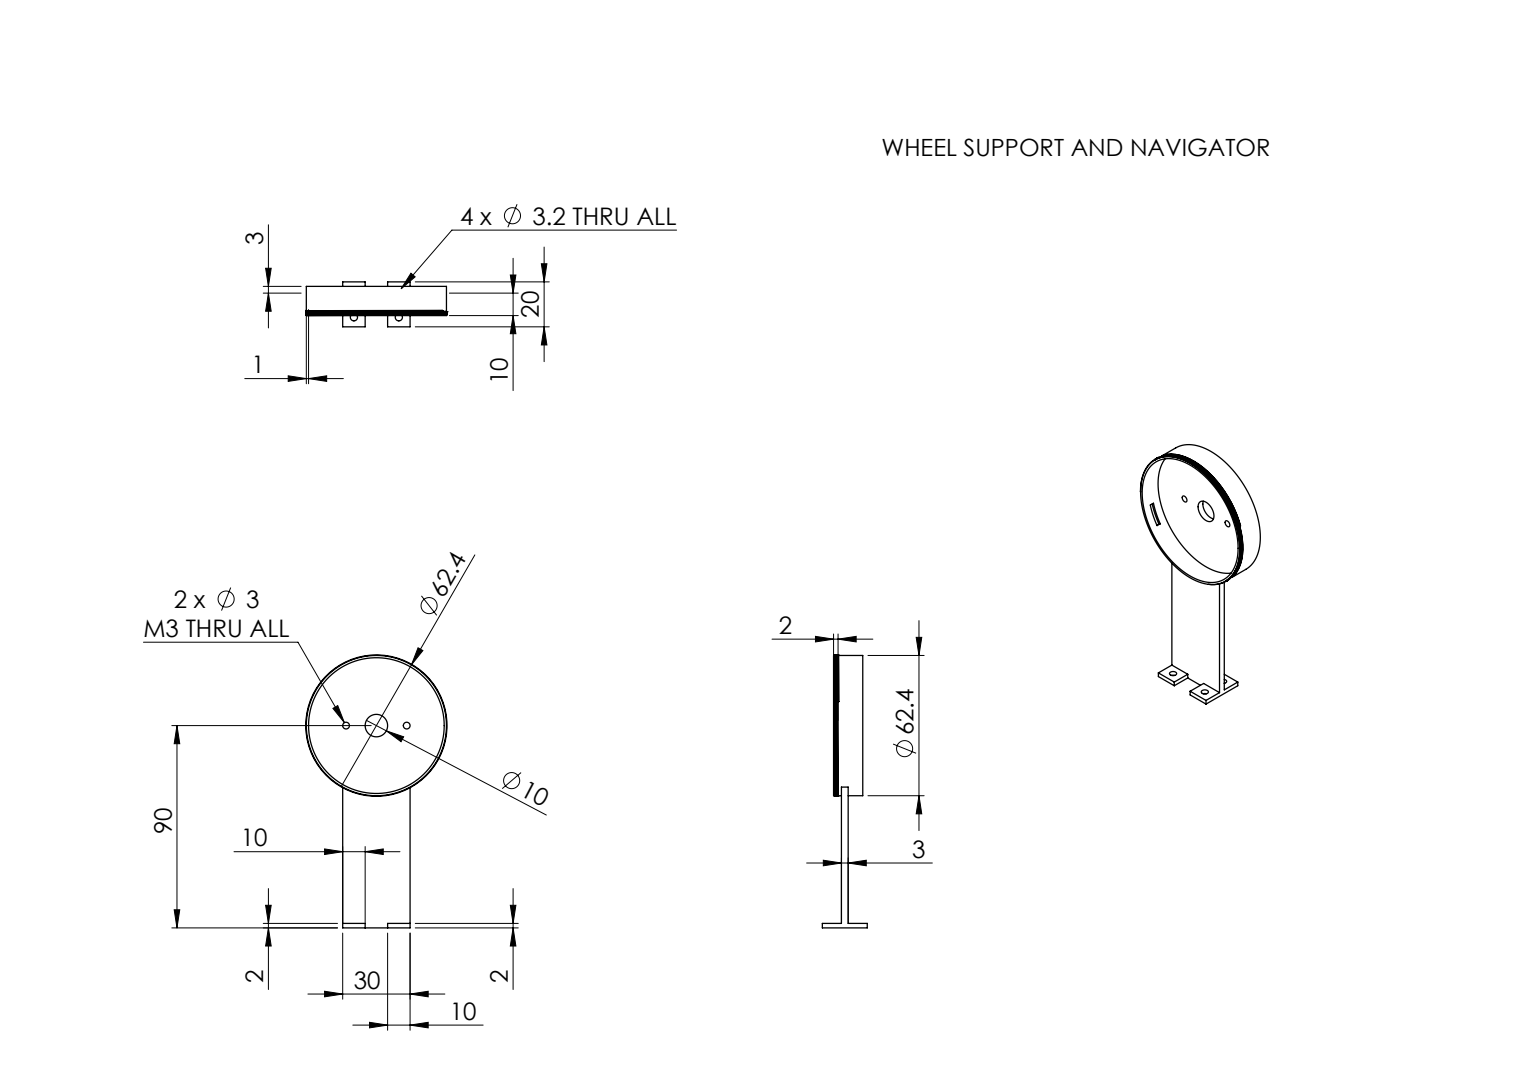
ISO-10303-21;
HEADER;
FILE_DESCRIPTION (('STEP AP214'),
    '1' );
FILE_NAME ('wheel support and navigator.step',
    '2026-10-26T05:17:54',
    ( '' ),
    ( '' ),
    'SwSTEP 2.0',
    'SolidWorks 2026',
    '' );
FILE_SCHEMA (( 'AUTOMOTIVE_DESIGN' ));
ENDSEC;

DATA;
#1=LINE ( 'NONE', #11989, #11081 ) ;
#2=CARTESIAN_POINT ( 'NONE',  ( 35.00000000000000000, 126.3079067962035822, 4.690625000614518036 ) ) ;
#5=AXIS2_PLACEMENT_3D ( 'NONE', #10923, #1108, #8837 ) ;
#14=CARTESIAN_POINT ( 'NONE',  ( 20.00000000000000355, 121.2009999999999934, -1.499999999999999556 ) ) ;
#18=ORIENTED_EDGE ( 'NONE', *, *, #2781, .T. ) ;
#24=LINE ( 'NONE', #4041, #9468 ) ;
#26=ORIENTED_EDGE ( 'NONE', *, *, #8182, .F. ) ;
#28=CARTESIAN_POINT ( 'NONE',  ( 46.99999999999995737, 90.00000000000000000, -8.000000000000000000 ) ) ;
#42=FACE_BOUND ( 'NONE', #647, .T. ) ;
#45=ORIENTED_EDGE ( 'NONE', *, *, #2569, .T. ) ;
#46=DIRECTION ( 'NONE',  ( 0.000000000000000000, -0.000000000000000000, -1.000000000000000000 ) ) ;
#54=AXIS2_PLACEMENT_3D ( 'NONE', #9236, #4147, #9107 ) ;
#61=( BOUNDED_CURVE ( )  B_SPLINE_CURVE ( 2, ( #6392, #1163, #3141, #10390, #7315, #302, #10192 ),
 .UNSPECIFIED., .F., .F. ) 
 B_SPLINE_CURVE_WITH_KNOTS ( ( 3, 2, 2, 3 ),
 ( 0.000000000000000000, 0.03333333333333339532, 0.06666666666666679064, 0.1000000000000001860 ),
 .UNSPECIFIED. ) 
 CURVE ( )  GEOMETRIC_REPRESENTATION_ITEM ( )  RATIONAL_B_SPLINE_CURVE ( ( 1.000000000000000000, 0.8660254037844387076, 1.000000000000000000, 0.8660254037844387076, 1.000000000000000000, 0.8660254037844380415, 1.000000000000000666 ) ) 
 REPRESENTATION_ITEM ( '' )  );
#62=CARTESIAN_POINT ( 'NONE',  ( 50.60000000000001563, 62.98000740192552627, 4.700000000000000178 ) ) ;
#84=DIRECTION ( 'NONE',  ( 2.891205793294679312E-17, 0.000000000000000000, -1.000000000000000000 ) ) ;
#91=AXIS2_PLACEMENT_3D ( 'NONE', #12672, #7630, #11620 ) ;
#108=VERTEX_POINT ( 'NONE', #7965 ) ;
#122=CARTESIAN_POINT ( 'NONE',  ( 35.00000000000000711, 53.97334320256736362, 3.425000001229034474 ) ) ;
#123=AXIS2_PLACEMENT_3D ( 'NONE', #3186, #84, #7099 ) ;
#127=CARTESIAN_POINT ( 'NONE',  ( 3.800000000000025135, 71.98667160128366049, 4.587500000000001243 ) ) ;
#134=CARTESIAN_POINT ( 'NONE',  ( 35.00000000000000000, 126.3079067962035822, 2.890625000614516882 ) ) ;
#144=DIRECTION ( 'NONE',  ( 0.000000000000000000, 0.000000000000000000, 1.000000000000000000 ) ) ;
#157=ORIENTED_EDGE ( 'NONE', *, *, #725, .T. ) ;
#158=CARTESIAN_POINT ( 'NONE',  ( 50.00000000000000000, 2.000000000000001776, 1.500000000000001332 ) ) ;
#173=DIRECTION ( 'NONE',  ( -0.000000000000000000, -0.000000000000000000, -1.000000000000000000 ) ) ;
#178=ORIENTED_EDGE ( 'NONE', *, *, #6430, .T. ) ;
#179=DIRECTION ( 'NONE',  ( 0.000000000000000000, 0.000000000000000000, 1.000000000000000000 ) ) ;
#189=ORIENTED_EDGE ( 'NONE', *, *, #6067, .T. ) ;
#190=CARTESIAN_POINT ( 'NONE',  ( 19.40000000000000924, 117.0199925980744666, 3.125000000000000000 ) ) ;
#193=VERTEX_POINT ( 'NONE', #2014 ) ;
#198=CARTESIAN_POINT ( 'NONE',  ( 3.556430356250028790, 71.84604660189818048, 3.940625000614518036 ) ) ;
#200=EDGE_CURVE ( 'NONE', #11286, #1104, #9001, .T. ) ;
#206=CARTESIAN_POINT ( 'NONE',  ( 66.19999999999988916, 71.98667160128361786, 3.950000001229034829 ) ) ;
#208=DIRECTION ( 'NONE',  ( -0.8660254037844365982, -0.5000000000000036637, 0.000000000000000000 ) ) ;
#245=DIRECTION ( 'NONE',  ( -1.000000000000000000, 0.000000000000000000, -0.000000000000000000 ) ) ;
#253=CARTESIAN_POINT ( 'NONE',  ( 35.00000000000000711, 53.97334320256736362, 3.762500000000000178 ) ) ;
#259=CYLINDRICAL_SURFACE ( 'NONE', #10517, 31.19999999999998863 ) ;
#264=CARTESIAN_POINT ( 'NONE',  ( 19.27821517812500574, 117.2309300971526937, 4.728125000614516793 ) ) ;
#265=CARTESIAN_POINT ( 'NONE',  ( 3.556430356250014579, 108.1539533981018053, 3.021875000614517415 ) ) ;
#268=STYLED_ITEM ( 'NONE', ( #1181 ), #2639 ) ;
#272=CARTESIAN_POINT ( 'NONE',  ( 12.66025403784434822, 85.80682368868758658, 1.000000000000000000 ) ) ;
#280=ORIENTED_EDGE ( 'NONE', *, *, #1510, .F. ) ;
#301=EDGE_CURVE ( 'NONE', #5352, #12120, #2388, .T. ) ;
#302=CARTESIAN_POINT ( 'NONE',  ( 66.20000000000005969, 108.0133283987162685, 4.475000001229034297 ) ) ;
#307=VERTEX_POINT ( 'NONE', #5210 ) ;
#313=CIRCLE ( 'NONE', #9312, 30.19999999999999218 ) ;
#316=VECTOR ( 'NONE', #11418, 1000.000000000000000 ) ;
#325=CARTESIAN_POINT ( 'NONE',  ( 3.556430356250015024, 90.00000000000000000, 4.859375000614517326 ) ) ;
#326=ORIENTED_EDGE ( 'NONE', *, *, #12262, .F. ) ;
#327=CARTESIAN_POINT ( 'NONE',  ( 5.011331584521381721, 81.39071625125095011, -1.000000000000000000 ) ) ;
#334=CARTESIAN_POINT ( 'NONE',  ( 50.72178482187499071, 117.2309300971526937, 2.909375000614517148 ) ) ;
#336=DIRECTION ( 'NONE',  ( 0.000000000000000000, 0.000000000000000000, 1.000000000000000000 ) ) ;
#346=ORIENTED_EDGE ( 'NONE', *, *, #1264, .T. ) ;
#361=CARTESIAN_POINT ( 'NONE',  ( 35.00000000000000000, 90.00000000000000000, -1.499999999999999556 ) ) ;
#368=ORIENTED_EDGE ( 'NONE', *, *, #2982, .T. ) ;
#389=PLANE ( 'NONE',  #10643 ) ;
#390=EDGE_CURVE ( 'NONE', #3842, #10632, #6639, .T. ) ;
#396=CARTESIAN_POINT ( 'NONE',  ( 19.27821517812503060, 62.76906990284727783, 3.134375000614517237 ) ) ;
#404=DIRECTION ( 'NONE',  ( 0.000000000000000000, 0.000000000000000000, -1.000000000000000000 ) ) ;
#414=DIRECTION ( 'NONE',  ( 0.000000000000000000, 0.000000000000000000, -1.000000000000000000 ) ) ;
#427=VERTEX_POINT ( 'NONE', #1412 ) ;
#435=CARTESIAN_POINT ( 'NONE',  ( 40.00000000000000000, 0.000000000000000000, 10.00000000000000000 ) ) ;
#450=PLANE ( 'NONE',  #6571 ) ;
#458=DIRECTION ( 'NONE',  ( 0.000000000000000000, -0.000000000000000000, 1.000000000000000000 ) ) ;
#460=CARTESIAN_POINT ( 'NONE',  ( 66.44356964375000985, 71.84604660189820891, 4.146875000614517859 ) ) ;
#461=CARTESIAN_POINT ( 'NONE',  ( 40.00000000000000000, 0.000000000000000000, -10.00000000000000000 ) ) ;
#471=ADVANCED_FACE ( 'NONE', ( #3454, #10443, #9457 ), #4494, .T. ) ;
#472=CARTESIAN_POINT ( 'NONE',  ( 35.00000000000000000, 90.00000000000000000, -8.000000000000000000 ) ) ;
#473=CARTESIAN_POINT ( 'NONE',  ( 35.00000000000000000, 126.0266567974326222, 4.887499999999999289 ) ) ;
#495=ORIENTED_EDGE ( 'NONE', *, *, #4508, .T. ) ;
#497=LINE ( 'NONE', #6524, #12081 ) ;
#503=DIRECTION ( 'NONE',  ( -0.000000000000000000, -0.000000000000000000, -1.000000000000000000 ) ) ;
#504=ORIENTED_EDGE ( 'NONE', *, *, #2993, .F. ) ;
#514=CARTESIAN_POINT ( 'NONE',  ( 66.19999999999988916, 71.98667160128361786, 4.287500000000000533 ) ) ;
#516=EDGE_CURVE ( 'NONE', #767, #10706, #9716, .T. ) ;
#519=CARTESIAN_POINT ( 'NONE',  ( 60.63303221600038739, 111.5086687461494392, 2.885734441893565538 ) ) ;
#523=VECTOR ( 'NONE', #11793, 1000.000000000000000 ) ;
#527=CARTESIAN_POINT ( 'NONE',  ( 3.800000000000015365, 90.00000000000000000, 4.100000000000000533 ) ) ;
#548=ADVANCED_FACE ( 'NONE', ( #11812, #12733 ), #8016, .F. ) ;
#550=DIRECTION ( 'NONE',  ( 0.000000000000000000, -1.000000000000000000, 0.000000000000000000 ) ) ;
#556=ADVANCED_FACE ( 'NONE', ( #3049, #10826 ), #5003, .F. ) ;
#574=CARTESIAN_POINT ( 'NONE',  ( 3.800000000000015365, 90.00000000000000000, 3.200000000000000178 ) ) ;
#586=CARTESIAN_POINT ( 'NONE',  ( 35.00000000000000711, 53.69209320379640360, 3.621875000614517059 ) ) ;
#588=PLANE ( 'NONE',  #11054 ) ;
#594=CARTESIAN_POINT ( 'NONE',  ( 66.20000000000004547, 108.0133283987162969, 3.912500000000000977 ) ) ;
#601=DIRECTION ( 'NONE',  ( -0.000000000000000000, 1.000000000000000000, -0.000000000000000000 ) ) ;
#611=ORIENTED_EDGE ( 'NONE', *, *, #2370, .T. ) ;
#621=CARTESIAN_POINT ( 'NONE',  ( 19.27821517812503060, 62.76906990284727783, 4.428125000614516971 ) ) ;
#633=ADVANCED_FACE ( 'NONE', ( #3905 ), #2920, .F. ) ;
#647=EDGE_LOOP ( 'NONE', ( #10608, #8614 ) ) ;
#651=CARTESIAN_POINT ( 'NONE',  ( 64.54728993811707483, 100.7543353701752125, 2.858851390224067313 ) ) ;
#652=EDGE_LOOP ( 'NONE', ( #3973, #10053 ) ) ;
#653=EDGE_CURVE ( 'NONE', #6728, #2032, #6175, .T. ) ;
#657=ORIENTED_EDGE ( 'NONE', *, *, #9994, .T. ) ;
#658=DIRECTION ( 'NONE',  ( 0.000000000000000000, -1.000000000000000000, 0.000000000000000000 ) ) ;
#662=CARTESIAN_POINT ( 'NONE',  ( 19.27821517812500574, 117.2309300971526937, 4.728125000614516793 ) ) ;
#664=DIRECTION ( 'NONE',  ( -0.000000000000000000, -0.000000000000000000, -1.000000000000000000 ) ) ;
#666=EDGE_CURVE ( 'NONE', #8482, #12120, #12330, .T. ) ;
#672=CARTESIAN_POINT ( 'NONE',  ( 66.44356964374998142, 108.1539533981018053, 3.771875000614516971 ) ) ;
#673=ORIENTED_EDGE ( 'NONE', *, *, #3401, .T. ) ;
#683=CARTESIAN_POINT ( 'NONE',  ( 66.44356964374998142, 108.1539533981018053, 3.715625000614517948 ) ) ;
#700=DIRECTION ( 'NONE',  ( 0.000000000000000000, 1.000000000000000000, 0.000000000000000000 ) ) ;
#704=CARTESIAN_POINT ( 'NONE',  ( 35.00000000000000000, 90.00000000000000000, -10.00000000000000000 ) ) ;
#709=LINE ( 'NONE', #2754, #11300 ) ;
#716=VERTEX_POINT ( 'NONE', #3314 ) ;
#725=EDGE_CURVE ( 'NONE', #12624, #3688, #9320, .T. ) ;
#730=CARTESIAN_POINT ( 'NONE',  ( 66.19999999999998863, 90.00000000000000000, 4.437500001229033764 ) ) ;
#735=CARTESIAN_POINT ( 'NONE',  ( 66.19999999999997442, 108.0133283987163253, 4.812500000000000000 ) ) ;
#739=EDGE_CURVE ( 'NONE', #5916, #6728, #5927, .T. ) ;
#741=CARTESIAN_POINT ( 'NONE',  ( 19.27821517812500574, 117.2309300971526937, 3.884375000614516793 ) ) ;
#742=ORIENTED_EDGE ( 'NONE', *, *, #6361, .T. ) ;
#752=CARTESIAN_POINT ( 'NONE',  ( 3.556430356250014579, 108.1539533981018053, 3.415625000614516793 ) ) ;
#756=EDGE_CURVE ( 'NONE', #5282, #3511, #6243, .T. ) ;
#759=ADVANCED_FACE ( 'NONE', ( #3115 ), #7095, .F. ) ;
#760=CIRCLE ( 'NONE', #2246, 1.500000000000001332 ) ;
#763=CARTESIAN_POINT ( 'NONE',  ( 19.40000000000000924, 117.0199925980744666, 4.474999999999999645 ) ) ;
#767=VERTEX_POINT ( 'NONE', #5128 ) ;
#768=LINE ( 'NONE', #8696, #9080 ) ;
#770=CIRCLE ( 'NONE', #12057, 1.599999999999997202 ) ;
#776=DIRECTION ( 'NONE',  ( -1.000000000000000000, 0.000000000000000000, 0.000000000000000000 ) ) ;
#786=CARTESIAN_POINT ( 'NONE',  ( 30.00000000000000711, 0.000000000000000000, -10.00000000000000000 ) ) ;
#787=DIRECTION ( 'NONE',  ( -1.000000000000000000, 0.000000000000000000, 0.000000000000000000 ) ) ;
#789=CARTESIAN_POINT ( 'NONE',  ( 35.00000000000000000, 126.0266567974326222, 4.550000001229034474 ) ) ;
#791=EDGE_CURVE ( 'NONE', #9339, #7595, #7229, .T. ) ;
#801=CARTESIAN_POINT ( 'NONE',  ( 3.556430356250015024, 90.00000000000000000, 4.859375000614517326 ) ) ;
#802=ORIENTED_EDGE ( 'NONE', *, *, #7272, .F. ) ;
#807=VECTOR ( 'NONE', #5449, 1000.000000000000000 ) ;
#810=VECTOR ( 'NONE', #8844, 1000.000000000000000 ) ;
#813=CARTESIAN_POINT ( 'NONE',  ( 35.00000000000000000, 126.3079067962036106, 4.240625000614517859 ) ) ;
#819=EDGE_LOOP ( 'NONE', ( #12547, #8502, #7527, #504 ) ) ;
#821=CARTESIAN_POINT ( 'NONE',  ( 35.00000000000000000, 90.00000000000000000, 5.000000000000000000 ) ) ;
#844=ORIENTED_EDGE ( 'NONE', *, *, #11090, .F. ) ;
#847=VECTOR ( 'NONE', #8727, 1000.000000000000000 ) ;
#852=CARTESIAN_POINT ( 'NONE',  ( 35.00000000000000000, 126.3079067962035822, 3.340625000614517059 ) ) ;
#855=ADVANCED_FACE ( 'NONE', ( #4477 ), #5384, .F. ) ;
#857=DIRECTION ( 'NONE',  ( -0.000000000000000000, -0.000000000000000000, -1.000000000000000000 ) ) ;
#862=VECTOR ( 'NONE', #12886, 1000.000000000000000 ) ;
#864=CARTESIAN_POINT ( 'NONE',  ( 35.00000000000000711, 53.69209320379640360, 4.071875000614516793 ) ) ;
#875=DIRECTION ( 'NONE',  ( 1.000000000000000000, 0.000000000000000000, 0.000000000000000000 ) ) ;
#890=CARTESIAN_POINT ( 'NONE',  ( 66.19999999999998863, 90.00000000000000000, 5.000000000000000000 ) ) ;
#892=VECTOR ( 'NONE', #11066, 1000.000000000000000 ) ;
#897=CARTESIAN_POINT ( 'NONE',  ( 50.00000000000000000, 62.64236852357281293, 1.500000000000001332 ) ) ;
#905=CARTESIAN_POINT ( 'NONE',  ( 35.00000000000000000, 90.00000000000000000, -1.000000000000000000 ) ) ;
#916=CARTESIAN_POINT ( 'NONE',  ( 19.27821517812503060, 62.76906990284727783, 3.978125000614516793 ) ) ;
#918=FACE_OUTER_BOUND ( 'NONE', #4746, .T. ) ;
#920=DIRECTION ( 'NONE',  ( -1.000000000000000000, 0.000000000000000000, 0.000000000000000000 ) ) ;
#929=CARTESIAN_POINT ( 'NONE',  ( 35.00000000000000711, 53.69209320379640360, 3.171875000614517326 ) ) ;
#930=ORIENTED_EDGE ( 'NONE', *, *, #4986, .T. ) ;
#932=CARTESIAN_POINT ( 'NONE',  ( 19.27821517812500574, 117.2309300971526937, 4.784375000614516260 ) ) ;
#933=DIRECTION ( 'NONE',  ( -0.000000000000000000, -0.000000000000000000, -1.000000000000000000 ) ) ;
#935=AXIS2_PLACEMENT_3D ( 'NONE', #9020, #5227, #4059 ) ;
#948=AXIS2_PLACEMENT_3D ( 'NONE', #2780, #4020, #9961 ) ;
#956=DIRECTION ( 'NONE',  ( -0.000000000000000000, 1.000000000000000000, -0.000000000000000000 ) ) ;
#958=DIRECTION ( 'NONE',  ( 0.000000000000000000, 0.000000000000000000, 1.000000000000000000 ) ) ;
#982=CARTESIAN_POINT ( 'NONE',  ( 66.44356964374999563, 90.00000000000000000, 4.128125000614517148 ) ) ;
#996=DIRECTION ( 'NONE',  ( -0.000000000000000000, -0.000000000000000000, -1.000000000000000000 ) ) ;
#997=CARTESIAN_POINT ( 'NONE',  ( 3.556430356250014579, 108.1539533981018053, 4.765625000614517326 ) ) ;
#1001=CIRCLE ( 'NONE', #4975, 1.599999999999997202 ) ;
#1006=CARTESIAN_POINT ( 'NONE',  ( 64.47099661891826372, 100.7265662098818098, 2.905726390019228056 ) ) ;
#1008=DIRECTION ( 'NONE',  ( -1.000000000000000000, 0.000000000000000000, 0.000000000000000000 ) ) ;
#1014=CARTESIAN_POINT ( 'NONE',  ( 3.800000000000015810, 108.0133283987162969, 3.612500000000000711 ) ) ;
#1015=CARTESIAN_POINT ( 'NONE',  ( 20.00000000000000355, 0.000000000000000000, -10.00000000000000000 ) ) ;
#1033=ORIENTED_EDGE ( 'NONE', *, *, #2858, .T. ) ;
#1036=CARTESIAN_POINT ( 'NONE',  ( 35.00000000000000000, 90.00000000000000000, -8.000000000000000000 ) ) ;
#1041=EDGE_LOOP ( 'NONE', ( #5551, #7064, #7845, #6591 ) ) ;
#1050=VERTEX_POINT ( 'NONE', #4863 ) ;
#1052=CARTESIAN_POINT ( 'NONE',  ( 66.19999999999998863, 90.00000000000000000, 4.774999999999999467 ) ) ;
#1059=CARTESIAN_POINT ( 'NONE',  ( 50.72178482187501203, 62.76906990284730625, 4.503125000614517148 ) ) ;
#1060=ORIENTED_EDGE ( 'NONE', *, *, #11229, .T. ) ;
#1061=CARTESIAN_POINT ( 'NONE',  ( 66.44356964374998142, 108.1539533981018053, 4.671875000614517326 ) ) ;
#1062=VECTOR ( 'NONE', #4789, 1000.000000000000000 ) ;
#1082=UNCERTAINTY_MEASURE_WITH_UNIT (LENGTH_MEASURE( 1.000000000000000082E-05 ), #4451, 'distance_accuracy_value', 'NONE');
#1089=ORIENTED_EDGE ( 'NONE', *, *, #8514, .F. ) ;
#1104=VERTEX_POINT ( 'NONE', #5047 ) ;
#1108=DIRECTION ( 'NONE',  ( -0.000000000000000000, -0.000000000000000000, -1.000000000000000000 ) ) ;
#1113=CARTESIAN_POINT ( 'NONE',  ( 17.66025403784438197, 77.14656965084323303, 1.000000000000000000 ) ) ;
#1116=CARTESIAN_POINT ( 'NONE',  ( 3.800000000000025135, 71.98667160128366049, 3.237500000000000266 ) ) ;
#1125=CARTESIAN_POINT ( 'NONE',  ( 3.556430356250015024, 90.00000000000000000, 4.353125000614517681 ) ) ;
#1130=VECTOR ( 'NONE', #208, 1000.000000000000000 ) ;
#1134=DIRECTION ( 'NONE',  ( 0.000000000000000000, 0.000000000000000000, 1.000000000000000000 ) ) ;
#1146=CIRCLE ( 'NONE', #2418, 1.599999999999990319 ) ;
#1152=CARTESIAN_POINT ( 'NONE',  ( 66.20000000000008811, 108.0133283987162542, 4.025000001229034119 ) ) ;
#1163=CARTESIAN_POINT ( 'NONE',  ( 3.800000000000015810, 108.0133283987162969, 4.625000001229034652 ) ) ;
#1167=DIRECTION ( 'NONE',  ( -1.000000000000000000, 0.000000000000000000, 0.000000000000000000 ) ) ;
#1179=CARTESIAN_POINT ( 'NONE',  ( 35.00000000000000000, 126.0266567974326222, 3.200000001229034385 ) ) ;
#1181=PRESENTATION_STYLE_ASSIGNMENT (( #10144 ) ) ;
#1185=CARTESIAN_POINT ( 'NONE',  ( 50.59999999999999432, 117.0199925980744666, 3.500000000000000444 ) ) ;
#1186=ORIENTED_EDGE ( 'NONE', *, *, #10214, .F. ) ;
#1189=CARTESIAN_POINT ( 'NONE',  ( 20.00000000000000355, 121.2009999999999934, 1.500000000000000444 ) ) ;
#1194=CARTESIAN_POINT ( 'NONE',  ( 66.44356964374998142, 108.1539533981018053, 4.165625000614516793 ) ) ;
#1196=CARTESIAN_POINT ( 'NONE',  ( 3.556430356250015024, 90.00000000000000000, 4.859375000614517326 ) ) ;
#1201=AXIS2_PLACEMENT_3D ( 'NONE', #8859, #2915, #336 ) ;
#1208=VECTOR ( 'NONE', #3192, 1000.000000000000000 ) ;
#1226=ORIENTED_EDGE ( 'NONE', *, *, #12302, .T. ) ;
#1230=EDGE_CURVE ( 'NONE', #5275, #1050, #1631, .T. ) ;
#1249=CARTESIAN_POINT ( 'NONE',  ( 66.19999999999998863, 90.00000000000000000, 3.087500001229034119 ) ) ;
#1252=ORIENTED_EDGE ( 'NONE', *, *, #1576, .T. ) ;
#1253=CARTESIAN_POINT ( 'NONE',  ( 50.59999999999999432, 117.0199925980744666, 4.400000000000000355 ) ) ;
#1256=ORIENTED_EDGE ( 'NONE', *, *, #8645, .T. ) ;
#1261=CARTESIAN_POINT ( 'NONE',  ( 3.556430356250014579, 108.1539533981018053, 4.315625000614517148 ) ) ;
#1262=CARTESIAN_POINT ( 'NONE',  ( 66.44356964375000985, 71.84604660189820891, 4.596875000614516260 ) ) ;
#1264=EDGE_CURVE ( 'NONE', #10380, #9690, #768, .T. ) ;
#1267=DIRECTION ( 'NONE',  ( 1.000000000000000000, 0.000000000000000000, -0.000000000000000000 ) ) ;
#1269=CARTESIAN_POINT ( 'NONE',  ( 50.00000000000000000, 0.000000000000000000, 10.00000000000000000 ) ) ;
#1285=LINE ( 'NONE', #7245, #3044 ) ;
#1287=EDGE_LOOP ( 'NONE', ( #8218, #2510 ) ) ;
#1308=CARTESIAN_POINT ( 'NONE',  ( 3.800000000000015365, 90.00000000000000000, 4.549999999999999822 ) ) ;
#1313=CARTESIAN_POINT ( 'NONE',  ( 3.556430356250014579, 108.1539533981018053, 4.371875000614517504 ) ) ;
#1316=DIRECTION ( 'NONE',  ( 0.000000000000000000, 0.000000000000000000, -1.000000000000000000 ) ) ;
#1331=EDGE_CURVE ( 'NONE', #307, #4218, #12687, .T. ) ;
#1334=CARTESIAN_POINT ( 'NONE',  ( 20.00000000000000355, 2.000000000000000000, 10.00000000000000000 ) ) ;
#1339=PRODUCT ( 'wheel support and navigator', 'wheel support and navigator', '', ( #4192 ) ) ;
#1342=ADVANCED_FACE ( 'NONE', ( #8575 ), #1756, .T. ) ;
#1346=ORIENTED_EDGE ( 'NONE', *, *, #2870, .F. ) ;
#1354=ORIENTED_EDGE ( 'NONE', *, *, #8514, .T. ) ;
#1362=AXIS2_PLACEMENT_3D ( 'NONE', #3082, #7982, #8050 ) ;
#1364=LINE ( 'NONE', #435, #5330 ) ;
#1368=CARTESIAN_POINT ( 'NONE',  ( 66.19999999999998863, 90.00000000000000000, 3.425000000000000266 ) ) ;
#1369=ORIENTED_EDGE ( 'NONE', *, *, #5464, .F. ) ;
#1373=AXIS2_PLACEMENT_3D ( 'NONE', #12342, #12472, #9393 ) ;
#1380=CARTESIAN_POINT ( 'NONE',  ( 50.72178482187501203, 62.76906990284730625, 3.659375000614517592 ) ) ;
#1382=EDGE_CURVE ( 'NONE', #5549, #3421, #6570, .T. ) ;
#1386=ORIENTED_EDGE ( 'NONE', *, *, #1264, .F. ) ;
#1390=CARTESIAN_POINT ( 'NONE',  ( 50.72178482187501203, 62.76906990284730625, 3.209375000614517415 ) ) ;
#1411=CARTESIAN_POINT ( 'NONE',  ( 20.00000000000000355, 2.000000000000000000, 10.00000000000000000 ) ) ;
#1412=CARTESIAN_POINT ( 'NONE',  ( 3.800000000000015365, 90.00000000000000000, 3.650000000000000355 ) ) ;
#1415=CARTESIAN_POINT ( 'NONE',  ( 50.72178482187499071, 117.2309300971526937, 4.653125000614517504 ) ) ;
#1420=ORIENTED_EDGE ( 'NONE', *, *, #6430, .F. ) ;
#1421=CARTESIAN_POINT ( 'NONE',  ( 30.00000000000000711, 0.000000000000000000, -1.499999999999999778 ) ) ;
#1422=LINE ( 'NONE', #7513, #9367 ) ;
#1425=EDGE_CURVE ( 'NONE', #10706, #1636, #1146, .T. ) ;
#1437=EDGE_CURVE ( 'NONE', #4511, #4278, #12939, .T. ) ;
#1454=DIRECTION ( 'NONE',  ( 0.000000000000000000, 0.000000000000000000, -1.000000000000000000 ) ) ;
#1456=CARTESIAN_POINT ( 'NONE',  ( 66.44356964374998142, 108.1539533981018053, 4.221875000614517148 ) ) ;
#1457=CARTESIAN_POINT ( 'NONE',  ( 35.00000000000000000, 126.3079067962035822, 4.690625000614518036 ) ) ;
#1468=CARTESIAN_POINT ( 'NONE',  ( 40.00000000000000000, 0.000000000000000000, -1.499999999999999778 ) ) ;
#1481=PLANE ( 'NONE',  #3567 ) ;
#1493=EDGE_LOOP ( 'NONE', ( #12432, #9531 ) ) ;
#1494=( BOUNDED_CURVE ( )  B_SPLINE_CURVE ( 2, ( #7440, #4369, #8360, #6386, #1415, #2473, #9461, #3522, #4498, #8491, #621, #12736, #4628, #5666, #3651, #813, #8616, #9719, #7631, #10828, #1807, #9784, #9656, #10766, #6774, #11683, #2668, #1872, #8803, #683, #4693, #12795, #3839, #3713, #4816, #7819, #2732, #752, #5793, #3776, #8739, #6643, #10638, #12607, #9595, #11815, #7757, #11747, #8679, #2862, #2793, #6835, #9847, #1680, #5857 ),
 .UNSPECIFIED., .F., .F. ) 
 B_SPLINE_CURVE_WITH_KNOTS ( ( 3, 2, 2, 2, 2, 2, 2, 2, 2, 2, 2, 2, 2, 2, 2, 2, 2, 2, 2, 2, 2, 2, 2, 2, 2, 2, 2, 3 ),
 ( 0.000000000000000000, 0.03333333333333333287, 0.06666666666666666574, 0.1000000000000000056, 0.1333333333333333315, 0.1666666666666666574, 0.2000000000000000111, 0.2333333333333333370, 0.2666666666666666630, 0.2999999999999999889, 0.3333333333333333148, 0.3666666666666666408, 0.4000000000000000222, 0.4333333333333333481, 0.4666666666666666741, 0.5000000000000000000, 0.5333333333333333259, 0.5666666666666666519, 0.5999999999999999778, 0.6333333333333333037, 0.6666666666666666297, 0.6999999999999999556, 0.7333333333333332815, 0.7666666666666667185, 0.8000000000000000444, 0.8333333333333333703, 0.8666666666666666963, 0.8887752010635167066 ),
 .UNSPECIFIED. ) 
 CURVE ( )  GEOMETRIC_REPRESENTATION_ITEM ( )  RATIONAL_B_SPLINE_CURVE ( ( 1.000000000000000000, 0.8660254037844387076, 1.000000000000000000, 0.8660254037844387076, 1.000000000000000000, 0.8660254037844387076, 1.000000000000000000, 0.8660254037844387076, 1.000000000000000000, 0.8660254037844387076, 1.000000000000000000, 0.8660254037844387076, 1.000000000000000000, 0.8660254037844387076, 1.000000000000000000, 0.8660254037844387076, 1.000000000000000000, 0.8660254037844387076, 1.000000000000000000, 0.8660254037844387076, 1.000000000000000000, 0.8660254037844387076, 1.000000000000000000, 0.8660254037844387076, 1.000000000000000000, 0.8660254037844387076, 1.000000000000000000, 0.8660254037844387076, 1.000000000000000000, 0.8660254037844387076, 1.000000000000000000, 0.8660254037844387076, 1.000000000000000000, 0.8660254037844387076, 1.000000000000000000, 0.8660254037844387076, 1.000000000000000000, 0.8660254037844387076, 1.000000000000000000, 0.8660254037844387076, 1.000000000000000000, 0.8660254037844387076, 1.000000000000000000, 0.8660254037844387076, 1.000000000000000000, 0.8660254037844387076, 1.000000000000000000, 0.8660254037844387076, 1.000000000000000000, 0.8660254037844387076, 1.000000000000000000, 0.8660254037844387076, 1.000000000000000000, 0.9111405409379251807, 0.9401542263054123438 ) ) 
 REPRESENTATION_ITEM ( '' )  );
#1495=ORIENTED_EDGE ( 'NONE', *, *, #10898, .T. ) ;
#1496=CARTESIAN_POINT ( 'NONE',  ( 21.49999999999998579, 90.00000000000000000, -8.000000000000000000 ) ) ;
#1501=CYLINDRICAL_SURFACE ( 'NONE', #12665, 4.999999999999997335 ) ;
#1509=ORIENTED_EDGE ( 'NONE', *, *, #5837, .T. ) ;
#1510=EDGE_CURVE ( 'NONE', #8482, #6635, #1285, .T. ) ;
#1511=CARTESIAN_POINT ( 'NONE',  ( 3.556430356250015024, 90.00000000000000000, 3.509375000614517681 ) ) ;
#1513=DIRECTION ( 'NONE',  ( 0.000000000000000000, -0.000000000000000000, -1.000000000000000000 ) ) ;
#1517=LINE ( 'NONE', #4602, #4637 ) ;
#1520=CARTESIAN_POINT ( 'NONE',  ( 19.27821517812500574, 117.2309300971526937, 3.884375000614516793 ) ) ;
#1521=CARTESIAN_POINT ( 'NONE',  ( 3.556430356250028790, 71.84604660189818048, 4.390625000614517326 ) ) ;
#1539=CARTESIAN_POINT ( 'NONE',  ( 40.00000000000000000, 90.00000000000000000, -10.00000000000000000 ) ) ;
#1557=CARTESIAN_POINT ( 'NONE',  ( 66.19999999999998863, 90.00000000000000000, 4.325000000000000178 ) ) ;
#1571=AXIS2_PLACEMENT_3D ( 'NONE', #11421, #4561, #11488 ) ;
#1574=DIRECTION ( 'NONE',  ( -0.000000000000000000, 1.000000000000000000, -0.000000000000000000 ) ) ;
#1576=EDGE_CURVE ( 'NONE', #3421, #5549, #7833, .T. ) ;
#1578=CARTESIAN_POINT ( 'NONE',  ( 35.00000000000000000, 126.3079067962035822, 2.946875000614516793 ) ) ;
#1594=LINE ( 'NONE', #12326, #8142 ) ;
#1608=VERTEX_POINT ( 'NONE', #158 ) ;
#1610=AXIS2_PLACEMENT_3D ( 'NONE', #8427, #11560, #5610 ) ;
#1615=DIRECTION ( 'NONE',  ( 0.000000000000000000, 0.000000000000000000, -1.000000000000000000 ) ) ;
#1616=ORIENTED_EDGE ( 'NONE', *, *, #8258, .F. ) ;
#1626=CARTESIAN_POINT ( 'NONE',  ( 3.800000000000015365, 90.00000000000000000, 4.549999999999999822 ) ) ;
#1631=LINE ( 'NONE', #9737, #9293 ) ;
#1634=VERTEX_POINT ( 'NONE', #3268 ) ;
#1636=VERTEX_POINT ( 'NONE', #3329 ) ;
#1645=CARTESIAN_POINT ( 'NONE',  ( 66.19999999999998863, 90.00000000000000000, 4.437500001229033764 ) ) ;
#1646=ORIENTED_EDGE ( 'NONE', *, *, #1230, .T. ) ;
#1653=CARTESIAN_POINT ( 'NONE',  ( 19.40000000000000924, 117.0199925980744666, 3.125000000000000000 ) ) ;
#1659=LINE ( 'NONE', #5581, #3550 ) ;
#1665=AXIS2_PLACEMENT_3D ( 'NONE', #9377, #9637, #4347 ) ;
#1673=AXIS2_PLACEMENT_3D ( 'NONE', #6725, #5686, #4896 ) ;
#1680=CARTESIAN_POINT ( 'NONE',  ( 60.63303222545420823, 111.5086687406912347, 2.829484441871016109 ) ) ;
#1681=VECTOR ( 'NONE', #5668, 1000.000000000000000 ) ;
#1683=CARTESIAN_POINT ( 'NONE',  ( 35.00000000000000000, 90.00000000000000000, -10.00000000000000000 ) ) ;
#1684=EDGE_LOOP ( 'NONE', ( #9223, #1947 ) ) ;
#1685=CARTESIAN_POINT ( 'NONE',  ( 20.00000000000000355, 2.000000000000000000, -10.00000000000000000 ) ) ;
#1687=EDGE_CURVE ( 'NONE', #11451, #7582, #12014, .T. ) ;
#1690=CIRCLE ( 'NONE', #3584, 30.19999999999999218 ) ;
#1697=DIRECTION ( 'NONE',  ( 0.000000000000000000, 1.000000000000000000, 0.000000000000000000 ) ) ;
#1699=EDGE_CURVE ( 'NONE', #8371, #11641, #8555, .T. ) ;
#1709=CARTESIAN_POINT ( 'NONE',  ( 30.00000000000000711, 2.000000000000000000, 10.00000000000000000 ) ) ;
#1717=CARTESIAN_POINT ( 'NONE',  ( 66.19999999999998863, 90.00000000000000000, 3.875000000000000000 ) ) ;
#1719=DIRECTION ( 'NONE',  ( -0.000000000000000000, 1.000000000000000000, -0.000000000000000000 ) ) ;
#1721=CARTESIAN_POINT ( 'NONE',  ( 35.00000000000000711, 53.69209320379640360, 4.015625000614517326 ) ) ;
#1731=CARTESIAN_POINT ( 'NONE',  ( 19.27821517812503060, 62.76906990284727783, 3.134375000614517237 ) ) ;
#1736=SURFACE_STYLE_FILL_AREA ( #6151 ) ;
#1739=CARTESIAN_POINT ( 'NONE',  ( 45.00000000000000000, 2.000000000000000000, 4.150000000000006573 ) ) ;
#1745=CARTESIAN_POINT ( 'NONE',  ( 5.904717470405908664, 81.90651283295660789, 5.000000000000000000 ) ) ;
#1747=AXIS2_PLACEMENT_3D ( 'NONE', #4106, #7242, #4302 ) ;
#1756=CYLINDRICAL_SURFACE ( 'NONE', #9711, 31.19999999999998863 ) ;
#1757=DIRECTION ( 'NONE',  ( -0.000000000000000000, -0.000000000000000000, -1.000000000000000000 ) ) ;
#1758=AXIS2_PLACEMENT_3D ( 'NONE', #7951, #4813, #9843 ) ;
#1771=ORIENTED_EDGE ( 'NONE', *, *, #9226, .T. ) ;
#1782=DIRECTION ( 'NONE',  ( 0.000000000000000000, 0.000000000000000000, 1.000000000000000000 ) ) ;
#1784=CARTESIAN_POINT ( 'NONE',  ( 3.800000000000015365, 90.00000000000000000, 4.212500001229034119 ) ) ;
#1790=CARTESIAN_POINT ( 'NONE',  ( 65.19999999999998863, 90.00000000000000000, 5.000000000000000000 ) ) ;
#1796=CARTESIAN_POINT ( 'NONE',  ( 19.27821517812500574, 117.2309300971526937, 4.334375000614516971 ) ) ;
#1802=ADVANCED_FACE ( 'NONE', ( #9532 ), #12606, .F. ) ;
#1807=CARTESIAN_POINT ( 'NONE',  ( 50.72178482187501203, 62.76906990284730625, 4.053125000614517859 ) ) ;
#1818=CARTESIAN_POINT ( 'NONE',  ( 20.00000000000000355, 2.000000000000000000, 10.00000000000000000 ) ) ;
#1820=DIRECTION ( 'NONE',  ( -2.891205793294679312E-17, -0.000000000000000000, 1.000000000000000000 ) ) ;
#1821=VERTEX_POINT ( 'NONE', #6707 ) ;
#1841=EDGE_CURVE ( 'NONE', #6922, #6635, #12237, .T. ) ;
#1848=CARTESIAN_POINT ( 'NONE',  ( 25.00000000000000355, 2.000000000000001332, 5.750000000000000000 ) ) ;
#1849=CARTESIAN_POINT ( 'NONE',  ( 19.40000000000002700, 62.98000740192551206, 3.837500001229034563 ) ) ;
#1858=ORIENTED_EDGE ( 'NONE', *, *, #10378, .T. ) ;
#1860=CARTESIAN_POINT ( 'NONE',  ( 19.27821517812503060, 62.76906990284727783, 4.484375000614516438 ) ) ;
#1865=FACE_OUTER_BOUND ( 'NONE', #5143, .T. ) ;
#1871=LINE ( 'NONE', #6773, #5335 ) ;
#1872=CARTESIAN_POINT ( 'NONE',  ( 35.00000000000000000, 126.3079067962036106, 3.790625000614517237 ) ) ;
#1873=LINE ( 'NONE', #7698, #1681 ) ;
#1876=ORIENTED_EDGE ( 'NONE', *, *, #8811, .T. ) ;
#1879=EDGE_LOOP ( 'NONE', ( #11841, #12494, #1646, #4523 ) ) ;
#1887=DIRECTION ( 'NONE',  ( 0.000000000000000000, 0.000000000000000000, 1.000000000000000000 ) ) ;
#1902=EDGE_CURVE ( 'NONE', #8617, #4915, #313, .T. ) ;
#1903=ORIENTED_EDGE ( 'NONE', *, *, #8109, .F. ) ;
#1909=CARTESIAN_POINT ( 'NONE',  ( 3.800000000000025580, 71.98667160128366049, 3.350000001229034297 ) ) ;
#1910=CARTESIAN_POINT ( 'NONE',  ( 19.27821517812500574, 117.2309300971526937, 3.828125000614516882 ) ) ;
#1911=EDGE_CURVE ( 'NONE', #6195, #5352, #1871, .T. ) ;
#1913=CARTESIAN_POINT ( 'NONE',  ( 35.00000000000000000, 90.00000000000000000, 5.000000000000000000 ) ) ;
#1915=( BOUNDED_CURVE ( )  B_SPLINE_CURVE ( 2, ( #1368, #4386, #7387, #5484, #9550, #9414, #574 ),
 .UNSPECIFIED., .F., .F. ) 
 B_SPLINE_CURVE_WITH_KNOTS ( ( 3, 2, 2, 3 ),
 ( 0.7000000000000001776, 0.7333333333333335036, 0.7666666666666669405, 0.8000000000000002665 ),
 .UNSPECIFIED. ) 
 CURVE ( )  GEOMETRIC_REPRESENTATION_ITEM ( )  RATIONAL_B_SPLINE_CURVE ( ( 0.9999999999999991118, 0.8660254037844395958, 1.000000000000000000, 0.8660254037844387076, 1.000000000000000000, 0.8660254037844378194, 1.000000000000000888 ) ) 
 REPRESENTATION_ITEM ( '' )  );
#1924=CARTESIAN_POINT ( 'NONE',  ( 50.72178482187501203, 62.76906990284730625, 3.209375000614517415 ) ) ;
#1929=EDGE_CURVE ( 'NONE', #6997, #4594, #6945, .T. ) ;
#1937=AXIS2_PLACEMENT_3D ( 'NONE', #12487, #3661, #12617 ) ;
#1941=CARTESIAN_POINT ( 'NONE',  ( 66.20000000000008811, 108.0133283987162542, 3.462499999999999467 ) ) ;
#1942=CARTESIAN_POINT ( 'NONE',  ( 45.00000000000000000, 0.000000000000000000, -4.150000000000003020 ) ) ;
#1946=DIRECTION ( 'NONE',  ( -0.8660254037844365982, -0.5000000000000036637, 0.000000000000000000 ) ) ;
#1947=ORIENTED_EDGE ( 'NONE', *, *, #9870, .T. ) ;
#1949=CARTESIAN_POINT ( 'NONE',  ( 30.00000000000000711, 121.2009999999999934, 1.500000000000000666 ) ) ;
#1954=LINE ( 'NONE', #12023, #12670 ) ;
#1960=DIRECTION ( 'NONE',  ( 1.000000000000000000, 0.000000000000000000, 0.000000000000000000 ) ) ;
#1965=ORIENTED_EDGE ( 'NONE', *, *, #3451, .F. ) ;
#1972=EDGE_LOOP ( 'NONE', ( #9502, #4976, #6099, #1965, #9834, #3104, #3537, #1858 ) ) ;
#1974=AXIS2_PLACEMENT_3D ( 'NONE', #7887, #5726, #5977 ) ;
#1977=CARTESIAN_POINT ( 'NONE',  ( 48.49999999999995737, 90.00000000000000000, -8.000000000000000000 ) ) ;
#1978=CARTESIAN_POINT ( 'NONE',  ( 66.19999999999997442, 108.0133283987163253, 4.025000001229034119 ) ) ;
#1991=CARTESIAN_POINT ( 'NONE',  ( 3.556430356250015024, 90.00000000000000000, 4.409375000614517148 ) ) ;
#1992=ORIENTED_EDGE ( 'NONE', *, *, #4002, .F. ) ;
#2004=VECTOR ( 'NONE', #10111, 1000.000000000000000 ) ;
#2008=DIRECTION ( 'NONE',  ( 0.000000000000000000, 0.000000000000000000, -1.000000000000000000 ) ) ;
#2009=ORIENTED_EDGE ( 'NONE', *, *, #12275, .T. ) ;
#2011=CIRCLE ( 'NONE', #3694, 31.19999999999999218 ) ;
#2014=CARTESIAN_POINT ( 'NONE',  ( 66.19999999999998863, 90.00000000000000000, 3.537500001229034297 ) ) ;
#2016=DIRECTION ( 'NONE',  ( 0.000000000000000000, 0.000000000000000000, 1.000000000000000000 ) ) ;
#2024=EDGE_LOOP ( 'NONE', ( #3519, #4907, #10756, #11768 ) ) ;
#2025=EDGE_CURVE ( 'NONE', #6338, #1104, #12661, .T. ) ;
#2027=DIRECTION ( 'NONE',  ( 0.000000000000000000, 0.000000000000000000, 1.000000000000000000 ) ) ;
#2030=VECTOR ( 'NONE', #7637, 1000.000000000000000 ) ;
#2032=VERTEX_POINT ( 'NONE', #5197 ) ;
#2035=EDGE_CURVE ( 'NONE', #4459, #5941, #9122, .T. ) ;
#2038=CARTESIAN_POINT ( 'NONE',  ( 19.99999999999998224, 90.00000000000000000, -8.000000000000000000 ) ) ;
#2044=( LENGTH_UNIT ( ) NAMED_UNIT ( * ) SI_UNIT ( .MILLI., .METRE. ) );
#2047=CARTESIAN_POINT ( 'NONE',  ( 35.00000000000000711, 53.97334320256736362, 4.212500000000000355 ) ) ;
#2056=CARTESIAN_POINT ( 'NONE',  ( 64.54728994471078352, 100.7543353520590870, 2.802601390178781404 ) ) ;
#2058=CARTESIAN_POINT ( 'NONE',  ( 35.00000000000000000, 126.3079067962036106, 4.746875000614517504 ) ) ;
#2078=CARTESIAN_POINT ( 'NONE',  ( 3.800000000000015365, 90.00000000000000000, 3.650000000000000355 ) ) ;
#2082=CARTESIAN_POINT ( 'NONE',  ( 25.00000000000000355, 2.000000000000000000, -7.349999999999991651 ) ) ;
#2084=ORIENTED_EDGE ( 'NONE', *, *, #11517, .F. ) ;
#2088=APPLICATION_CONTEXT ( 'automotive_design' ) ;
#2092=CARTESIAN_POINT ( 'NONE',  ( 64.54728994471078352, 100.7543353520590870, 2.802601390178781404 ) ) ;
#2093=ORIENTED_EDGE ( 'NONE', *, *, #7600, .T. ) ;
#2095=AXIS2_PLACEMENT_3D ( 'NONE', #2749, #4771, #1887 ) ;
#2101=VERTEX_POINT ( 'NONE', #7161 ) ;
#2109=CARTESIAN_POINT ( 'NONE',  ( 3.800000000000025135, 71.98667160128366049, 3.800000001229034030 ) ) ;
#2113=CARTESIAN_POINT ( 'NONE',  ( 66.44356964374998142, 108.1539533981018053, 4.671875000614516438 ) ) ;
#2115=CARTESIAN_POINT ( 'NONE',  ( 25.00000000000000355, 0.000000000000000000, -5.750000000000000000 ) ) ;
#2122=CARTESIAN_POINT ( 'NONE',  ( 50.72178482187501203, 62.76906990284730625, 3.603125000614517681 ) ) ;
#2126=CARTESIAN_POINT ( 'NONE',  ( 40.00000000000000000, 2.000000000000000000, -1.499999999999999556 ) ) ;
#2140=LINE ( 'NONE', #7241, #1208 ) ;
#2144=ORIENTED_EDGE ( 'NONE', *, *, #653, .T. ) ;
#2149=( BOUNDED_SURFACE ( )  B_SPLINE_SURFACE ( 1, 2, ( 
 ( #801, #2721, #6694, #9836, #11929, #7808, #2974, #11865, #10752, #7878, #1860, #12785, #1991, #9897, #1796, #10939, #5847, #8666, #12914, #8854, #5969, #864, #3828, #12662, #6955, #4934, #741, #4867, #5718, #672, #12850, #2783, #3898, #3704, #6891, #7685, #5782, #10879, #11804, #11670, #7746, #6823, #11733, #10690, #1924, #929, #1731, #9705, #4741, #8728, #12723, #3764, #6761, #9772, #4806 ),
 ( #6098, #997, #264, #2, #3106, #3038, #4023, #7219, #1059, #7022, #5186, #2259, #1125, #1261, #3306, #11003, #8008, #1194, #4995, #7088, #6235, #10159, #12189, #198, #2322, #11070, #9175, #4216, #11990, #10225, #9044, #8203, #2122, #3239, #10089, #8979, #5119, #11133, #9110, #3173, #6035, #8073, #11206, #10029, #4086, #6166, #5253, #9966, #12060, #9241, #4281, #134, #8269, #12258, #2056 ) ),
 .UNSPECIFIED., .F., .F., .F. ) 
 B_SPLINE_SURFACE_WITH_KNOTS ( ( 2, 2 ),
 ( 3, 2, 2, 2, 2, 2, 2, 2, 2, 2, 2, 2, 2, 2, 2, 2, 2, 2, 2, 2, 2, 2, 2, 2, 2, 2, 2, 3 ),
 ( 0.000000000000000000, 1.000000000000000000 ),
 ( 0.000000000000000000, 0.03333333333333333287, 0.06666666666666666574, 0.1000000000000000056, 0.1333333333333333315, 0.1666666666666666574, 0.2000000000000000111, 0.2333333333333333370, 0.2666666666666666630, 0.2999999999999999889, 0.3333333333333333148, 0.3666666666666666408, 0.4000000000000000222, 0.4333333333333333481, 0.4666666666666666741, 0.5000000000000000000, 0.5333333333333333259, 0.5666666666666666519, 0.5999999999999999778, 0.6333333333333333037, 0.6666666666666666297, 0.6999999999999999556, 0.7333333333333332815, 0.7666666666666667185, 0.8000000000000000444, 0.8333333333333333703, 0.8666666666666666963, 0.8887752010635167066 ),
 .UNSPECIFIED. ) 
 GEOMETRIC_REPRESENTATION_ITEM ( )  RATIONAL_B_SPLINE_SURFACE ( (
 ( 1.000000000000000000, 0.8660254037844387076, 1.000000000000000000, 0.8660254037844387076, 1.000000000000000000, 0.8660254037844387076, 1.000000000000000000, 0.8660254037844387076, 1.000000000000000000, 0.8660254037844387076, 1.000000000000000000, 0.8660254037844387076, 1.000000000000000000, 0.8660254037844387076, 1.000000000000000000, 0.8660254037844387076, 1.000000000000000000, 0.8660254037844387076, 1.000000000000000000, 0.8660254037844387076, 1.000000000000000000, 0.8660254037844387076, 1.000000000000000000, 0.8660254037844387076, 1.000000000000000000, 0.8660254037844387076, 1.000000000000000000, 0.8660254037844387076, 1.000000000000000000, 0.8660254037844387076, 1.000000000000000000, 0.8660254037844387076, 1.000000000000000000, 0.8660254037844387076, 1.000000000000000000, 0.8660254037844387076, 1.000000000000000000, 0.8660254037844387076, 1.000000000000000000, 0.8660254037844387076, 1.000000000000000000, 0.8660254037844387076, 1.000000000000000000, 0.8660254037844387076, 1.000000000000000000, 0.8660254037844387076, 1.000000000000000000, 0.8660254037844387076, 1.000000000000000000, 0.8660254037844387076, 1.000000000000000000, 0.8660254037844387076, 1.000000000000000000, 0.9111405409379251807, 0.9401542263054123438),
 ( 1.000000000000000000, 0.8660254037844387076, 1.000000000000000000, 0.8660254037844387076, 1.000000000000000000, 0.8660254037844387076, 1.000000000000000000, 0.8660254037844387076, 1.000000000000000000, 0.8660254037844387076, 1.000000000000000000, 0.8660254037844387076, 1.000000000000000000, 0.8660254037844387076, 1.000000000000000000, 0.8660254037844387076, 1.000000000000000000, 0.8660254037844387076, 1.000000000000000000, 0.8660254037844387076, 1.000000000000000000, 0.8660254037844387076, 1.000000000000000000, 0.8660254037844387076, 1.000000000000000000, 0.8660254037844387076, 1.000000000000000000, 0.8660254037844387076, 1.000000000000000000, 0.8660254037844387076, 1.000000000000000000, 0.8660254037844387076, 1.000000000000000000, 0.8660254037844387076, 1.000000000000000000, 0.8660254037844387076, 1.000000000000000000, 0.8660254037844387076, 1.000000000000000000, 0.8660254037844387076, 1.000000000000000000, 0.8660254037844387076, 1.000000000000000000, 0.8660254037844387076, 1.000000000000000000, 0.8660254037844387076, 1.000000000000000000, 0.8660254037844387076, 1.000000000000000000, 0.8660254037844387076, 1.000000000000000000, 0.8660254037844387076, 1.000000000000000000, 0.9111405409379251807, 0.9401542263054123438) ) ) 
 REPRESENTATION_ITEM ( '' )  SURFACE ( )  );
#2153=CARTESIAN_POINT ( 'NONE',  ( 20.00000000000000355, 2.000000000000001776, 1.500000000000000444 ) ) ;
#2179=CARTESIAN_POINT ( 'NONE',  ( 3.800000000000025135, 71.98667160128366049, 4.137500000000001066 ) ) ;
#2184=AXIS2_PLACEMENT_3D ( 'NONE', #4876, #10697, #2791 ) ;
#2188=DIRECTION ( 'NONE',  ( 0.000000000000000000, 0.000000000000000000, 1.000000000000000000 ) ) ;
#2190=VERTEX_POINT ( 'NONE', #10493 ) ;
#2208=ORIENTED_EDGE ( 'NONE', *, *, #7500, .T. ) ;
#2210=DIRECTION ( 'NONE',  ( -1.000000000000000000, 0.000000000000000000, 0.000000000000000000 ) ) ;
#2223=EDGE_CURVE ( 'NONE', #3511, #12839, #2429, .T. ) ;
#2230=ORIENTED_EDGE ( 'NONE', *, *, #7511, .F. ) ;
#2246=AXIS2_PLACEMENT_3D ( 'NONE', #5889, #9882, #787 ) ;
#2251=CARTESIAN_POINT ( 'NONE',  ( 19.40000000000002700, 62.98000740192551206, 3.275000000000000355 ) ) ;
#2257=LINE ( 'NONE', #3238, #4625 ) ;
#2259=CARTESIAN_POINT ( 'NONE',  ( 3.556430356250028790, 71.84604660189818048, 4.390625000614517326 ) ) ;
#2260=CARTESIAN_POINT ( 'NONE',  ( 19.27821517812500574, 117.2309300971526937, 4.334375000614516971 ) ) ;
#2266=DIRECTION ( 'NONE',  ( -0.000000000000000000, 1.000000000000000000, -0.000000000000000000 ) ) ;
#2268=CARTESIAN_POINT ( 'NONE',  ( 45.00000000000000000, 2.000000000000001332, -5.750000000000000000 ) ) ;
#2270=CARTESIAN_POINT ( 'NONE',  ( 3.800000000000015365, 90.00000000000000000, 5.000000000000000000 ) ) ;
#2278=DIRECTION ( 'NONE',  ( 0.000000000000000000, 0.000000000000000000, 1.000000000000000000 ) ) ;
#2280=VECTOR ( 'NONE', #12698, 1000.000000000000000 ) ;
#2296=VECTOR ( 'NONE', #8196, 1000.000000000000000 ) ;
#2297=CYLINDRICAL_SURFACE ( 'NONE', #2832, 1.500000000000001332 ) ;
#2309=CARTESIAN_POINT ( 'NONE',  ( 3.800000000000015365, 108.0133283987163111, 3.275000001229034119 ) ) ;
#2313=CARTESIAN_POINT ( 'NONE',  ( 3.800000000000015365, 90.00000000000000000, 4.100000000000000533 ) ) ;
#2315=LINE ( 'NONE', #6351, #2296 ) ;
#2322=CARTESIAN_POINT ( 'NONE',  ( 3.556430356250015024, 90.00000000000000000, 3.903125000614517504 ) ) ;
#2324=CARTESIAN_POINT ( 'NONE',  ( 50.72178482187501203, 62.76906990284730625, 4.109375000614517326 ) ) ;
#2325=CARTESIAN_POINT ( 'NONE',  ( 40.00000000000000000, 0.000000000000000000, 10.00000000000000000 ) ) ;
#2329=CARTESIAN_POINT ( 'NONE',  ( 45.00000000000000000, 2.000000000000000000, -5.750000000000000000 ) ) ;
#2336=EDGE_CURVE ( 'NONE', #7731, #6997, #11965, .T. ) ;
#2340=LINE ( 'NONE', #4364, #2004 ) ;
#2345=ORIENTED_EDGE ( 'NONE', *, *, #2733, .F. ) ;
#2350=ORIENTED_EDGE ( 'NONE', *, *, #3130, .T. ) ;
#2370=EDGE_CURVE ( 'NONE', #11848, #9339, #5779, .T. ) ;
#2373=DIRECTION ( 'NONE',  ( -0.3420201803727477285, 0.9396926073018736503, 0.000000000000000000 ) ) ;
#2383=CARTESIAN_POINT ( 'NONE',  ( 3.556430356250015024, 90.00000000000000000, 3.959375000614517415 ) ) ;
#2388=CIRCLE ( 'NONE', #12400, 31.19999999999999218 ) ;
#2395=ORIENTED_EDGE ( 'NONE', *, *, #2605, .F. ) ;
#2396=ADVANCED_FACE ( 'NONE', ( #3762 ), #7744, .T. ) ;
#2418=AXIS2_PLACEMENT_3D ( 'NONE', #6060, #956, #2016 ) ;
#2423=VERTEX_POINT ( 'NONE', #11987 ) ;
#2424=DIRECTION ( 'NONE',  ( -1.000000000000000000, 0.000000000000000000, 0.000000000000000000 ) ) ;
#2425=ORIENTED_EDGE ( 'NONE', *, *, #7142, .T. ) ;
#2429=CIRCLE ( 'NONE', #9729, 31.20000000000000284 ) ;
#2437=DIRECTION ( 'NONE',  ( 0.000000000000000000, 0.000000000000000000, 1.000000000000000000 ) ) ;
#2441=CARTESIAN_POINT ( 'NONE',  ( 64.43284985331906967, 100.7126819209670145, 2.929163888449521025 ) ) ;
#2442=ORIENTED_EDGE ( 'NONE', *, *, #10214, .T. ) ;
#2443=DIRECTION ( 'NONE',  ( 0.000000000000000000, -1.000000000000000000, 0.000000000000000000 ) ) ;
#2450=CARTESIAN_POINT ( 'NONE',  ( 35.00000000000000000, 126.3079067962036106, 3.846875000614517592 ) ) ;
#2452=DIRECTION ( 'NONE',  ( 0.000000000000000000, 0.000000000000000000, 1.000000000000000000 ) ) ;
#2458=AXIS2_PLACEMENT_3D ( 'NONE', #11881, #2008, #10893 ) ;
#2465=ORIENTED_EDGE ( 'NONE', *, *, #12549, .F. ) ;
#2473=CARTESIAN_POINT ( 'NONE',  ( 66.44356964374998142, 108.1539533981018053, 4.615625000614516971 ) ) ;
#2478=EDGE_LOOP ( 'NONE', ( #5655, #9956 ) ) ;
#2481=EDGE_CURVE ( 'NONE', #2101, #4251, #4211, .T. ) ;
#2489=ADVANCED_FACE ( 'NONE', ( #12122 ), #259, .T. ) ;
#2504=CARTESIAN_POINT ( 'NONE',  ( 19.27821517812500574, 117.2309300971526937, 3.884375000614516793 ) ) ;
#2510=ORIENTED_EDGE ( 'NONE', *, *, #1576, .F. ) ;
#2513=CARTESIAN_POINT ( 'NONE',  ( 3.556430356250028790, 71.84604660189818048, 3.096875000614517148 ) ) ;
#2514=CARTESIAN_POINT ( 'NONE',  ( 50.72178482187501203, 62.76906990284730625, 4.503125000614517148 ) ) ;
#2524=CARTESIAN_POINT ( 'NONE',  ( 66.20000000000005969, 108.0133283987162685, 4.812499999999999112 ) ) ;
#2530=ORIENTED_EDGE ( 'NONE', *, *, #6268, .T. ) ;
#2531=ADVANCED_FACE ( 'NONE', ( #8070 ), #7146, .F. ) ;
#2532=EDGE_CURVE ( 'NONE', #4396, #427, #3068, .T. ) ;
#2533=CARTESIAN_POINT ( 'NONE',  ( 50.00000000000000000, 2.000000000000000000, 10.00000000000000000 ) ) ;
#2558=ORIENTED_EDGE ( 'NONE', *, *, #2882, .F. ) ;
#2563=AXIS2_PLACEMENT_3D ( 'NONE', #1848, #1719, #3692 ) ;
#2565=CARTESIAN_POINT ( 'NONE',  ( 3.556430356250014579, 108.1539533981018053, 3.921875000614517326 ) ) ;
#2566=ORIENTED_EDGE ( 'NONE', *, *, #6741, .F. ) ;
#2569=EDGE_CURVE ( 'NONE', #3421, #12815, #9041, .T. ) ;
#2583=VECTOR ( 'NONE', #3302, 1000.000000000000000 ) ;
#2605=EDGE_CURVE ( 'NONE', #3551, #10547, #11766, .T. ) ;
#2608=CARTESIAN_POINT ( 'NONE',  ( 35.00000000000000000, 90.00000000000000000, 5.000000000000000000 ) ) ;
#2609=ORIENTED_EDGE ( 'NONE', *, *, #9479, .F. ) ;
#2614=ORIENTED_EDGE ( 'NONE', *, *, #7142, .F. ) ;
#2623=FACE_OUTER_BOUND ( 'NONE', #6598, .T. ) ;
#2632=CARTESIAN_POINT ( 'NONE',  ( 66.44356964374998142, 108.1539533981018053, 4.221875000614517148 ) ) ;
#2634=VECTOR ( 'NONE', #12268, 1000.000000000000000 ) ;
#2639=ADVANCED_BREP_SHAPE_REPRESENTATION ( '', ( #3242, #5704 ), #11354 ) ;
#2643=CARTESIAN_POINT ( 'NONE',  ( 50.59999999999999432, 117.0199925980744666, 3.050000000000000266 ) ) ;
#2656=LINE ( 'NONE', #2720, #10467 ) ;
#2665=CARTESIAN_POINT ( 'NONE',  ( 20.00000000000000355, 0.000000000000000000, 10.00000000000000000 ) ) ;
#2668=CARTESIAN_POINT ( 'NONE',  ( 19.27821517812500574, 117.2309300971526937, 3.828125000614516882 ) ) ;
#2670=FACE_OUTER_BOUND ( 'NONE', #3257, .T. ) ;
#2671=ORIENTED_EDGE ( 'NONE', *, *, #1841, .T. ) ;
#2684=LINE ( 'NONE', #1949, #10025 ) ;
#2693=DIRECTION ( 'NONE',  ( 0.000000000000000000, 0.000000000000000000, -1.000000000000000000 ) ) ;
#2701=CARTESIAN_POINT ( 'NONE',  ( 50.60000000000001563, 62.98000740192552627, 3.012500001229034829 ) ) ;
#2705=ORIENTED_EDGE ( 'NONE', *, *, #9543, .T. ) ;
#2707=CARTESIAN_POINT ( 'NONE',  ( 60.43447303579327468, 111.3420569435211149, 3.026359439817805086 ) ) ;
#2709=VECTOR ( 'NONE', #6817, 1000.000000000000000 ) ;
#2710=CARTESIAN_POINT ( 'NONE',  ( 35.00000000000000711, 53.69209320379640360, 3.565625000614517592 ) ) ;
#2712=CIRCLE ( 'NONE', #3755, 1.599999999999997202 ) ;
#2713=CYLINDRICAL_SURFACE ( 'NONE', #3339, 31.19999999999998863 ) ;
#2714=CARTESIAN_POINT ( 'NONE',  ( 35.00000000000000711, 53.97334320256736362, 3.875000001229034208 ) ) ;
#2720=CARTESIAN_POINT ( 'NONE',  ( 3.678215178125014972, 90.00000000000000000, 4.732812500921776078 ) ) ;
#2721=CARTESIAN_POINT ( 'NONE',  ( 3.556430356250014579, 108.1539533981018053, 4.821875000614516793 ) ) ;
#2725=ORIENTED_EDGE ( 'NONE', *, *, #9994, .F. ) ;
#2731=ADVANCED_FACE ( 'NONE', ( #4005 ), #5036, .F. ) ;
#2732=CARTESIAN_POINT ( 'NONE',  ( 3.556430356250015024, 90.00000000000000000, 3.453125000614517770 ) ) ;
#2733=EDGE_CURVE ( 'NONE', #5916, #10118, #4195, .T. ) ;
#2744=DIRECTION ( 'NONE',  ( -0.000000000000000000, -0.000000000000000000, -1.000000000000000000 ) ) ;
#2747=ORIENTED_EDGE ( 'NONE', *, *, #12032, .F. ) ;
#2749=CARTESIAN_POINT ( 'NONE',  ( 45.00000000000000000, 0.000000000000000000, -5.750000000000000000 ) ) ;
#2751=DIRECTION ( 'NONE',  ( 1.000000000000000000, 0.000000000000000000, 0.000000000000000000 ) ) ;
#2754=CARTESIAN_POINT ( 'NONE',  ( 17.66025403784438197, 77.14656965084323303, -1.000000000000000000 ) ) ;
#2756=ADVANCED_FACE ( 'NONE', ( #6140, #10204 ), #5097, .F. ) ;
#2770=CARTESIAN_POINT ( 'NONE',  ( 45.00000000000000000, 0.000000000000000000, -7.349999999999996980 ) ) ;
#2774=CARTESIAN_POINT ( 'NONE',  ( 66.19999999999997442, 108.0133283987163253, 4.475000001229034297 ) ) ;
#2780=CARTESIAN_POINT ( 'NONE',  ( 35.00000000000000000, 90.00000000000000000, 5.000000000000000000 ) ) ;
#2781=EDGE_CURVE ( 'NONE', #10632, #307, #24, .T. ) ;
#2782=DIRECTION ( 'NONE',  ( 1.000000000000000000, 0.000000000000000000, 0.000000000000000000 ) ) ;
#2783=CARTESIAN_POINT ( 'NONE',  ( 66.44356964374999563, 71.84604660189820891, 3.696875000614517237 ) ) ;
#2791=DIRECTION ( 'NONE',  ( -1.000000000000000000, 0.000000000000000000, 0.000000000000000000 ) ) ;
#2793=CARTESIAN_POINT ( 'NONE',  ( 19.27821517812500574, 117.2309300971526937, 2.928125000614517415 ) ) ;
#2794=EDGE_CURVE ( 'NONE', #3842, #4251, #11757, .T. ) ;
#2802=EDGE_CURVE ( 'NONE', #4594, #11781, #10838, .T. ) ;
#2805=DIRECTION ( 'NONE',  ( 1.000000000000000000, -0.000000000000000000, 0.000000000000000000 ) ) ;
#2806=CARTESIAN_POINT ( 'NONE',  ( 3.678215178125014972, 90.00000000000000000, 4.929687500307258219 ) ) ;
#2812=FACE_OUTER_BOUND ( 'NONE', #12565, .T. ) ;
#2817=VERTEX_POINT ( 'NONE', #9856 ) ;
#2819=VERTEX_POINT ( 'NONE', #1942 ) ;
#2826=EDGE_CURVE ( 'NONE', #5941, #3688, #7832, .T. ) ;
#2832=AXIS2_PLACEMENT_3D ( 'NONE', #10199, #173, #1167 ) ;
#2833=DIRECTION ( 'NONE',  ( -0.000000000000000000, 1.000000000000000000, -0.000000000000000000 ) ) ;
#2836=CARTESIAN_POINT ( 'NONE',  ( 50.60000000000001563, 62.98000740192552627, 3.912500001229034297 ) ) ;
#2839=DIRECTION ( 'NONE',  ( -1.000000000000000000, 0.000000000000000000, 0.000000000000000000 ) ) ;
#2841=( BOUNDED_CURVE ( )  B_SPLINE_CURVE ( 2, ( #527, #6488, #5769, #11657, #12649, #594, #1717 ),
 .UNSPECIFIED., .F., .F. ) 
 B_SPLINE_CURVE_WITH_KNOTS ( ( 3, 2, 2, 3 ),
 ( 0.3999999999999999667, 0.4333333333333333481, 0.4666666666666667296, 0.5000000000000001110 ),
 .UNSPECIFIED. ) 
 CURVE ( )  GEOMETRIC_REPRESENTATION_ITEM ( )  RATIONAL_B_SPLINE_CURVE ( ( 1.000000000000000444, 0.8660254037844385966, 1.000000000000000000, 0.8660254037844387076, 1.000000000000000000, 0.8660254037844382635, 1.000000000000000444 ) ) 
 REPRESENTATION_ITEM ( '' )  );
#2851=EDGE_LOOP ( 'NONE', ( #11355, #4320, #9624, #10703 ) ) ;
#2858=EDGE_CURVE ( 'NONE', #6325, #1821, #8876, .T. ) ;
#2862=CARTESIAN_POINT ( 'NONE',  ( 3.556430356250014579, 108.1539533981018053, 2.965625000614517504 ) ) ;
#2864=DIRECTION ( 'NONE',  ( -0.000000000000000000, -1.000000000000000000, -0.000000000000000000 ) ) ;
#2870=EDGE_CURVE ( 'NONE', #2423, #2817, #6718, .T. ) ;
#2874=LINE ( 'NONE', #9609, #3365 ) ;
#2876=DIRECTION ( 'NONE',  ( -0.000000000000000000, 1.000000000000000000, -0.000000000000000000 ) ) ;
#2879=ORIENTED_EDGE ( 'NONE', *, *, #9817, .T. ) ;
#2881=ORIENTED_EDGE ( 'NONE', *, *, #4201, .T. ) ;
#2882=EDGE_CURVE ( 'NONE', #12839, #3511, #6115, .T. ) ;
#2890=EDGE_LOOP ( 'NONE', ( #12441, #3402, #12951, #5471 ) ) ;
#2895=EDGE_LOOP ( 'NONE', ( #1089, #6800 ) ) ;
#2901=CARTESIAN_POINT ( 'NONE',  ( 50.72178482187499071, 117.2309300971526937, 2.853125000614517237 ) ) ;
#2905=FACE_OUTER_BOUND ( 'NONE', #9710, .T. ) ;
#2915=DIRECTION ( 'NONE',  ( -0.000000000000000000, 1.000000000000000000, -0.000000000000000000 ) ) ;
#2920=CYLINDRICAL_SURFACE ( 'NONE', #12831, 1.599999999999993872 ) ;
#2921=AXIS2_PLACEMENT_3D ( 'NONE', #9697, #11792, #2839 ) ;
#2926=EDGE_CURVE ( 'NONE', #9339, #1634, #6783, .T. ) ;
#2931=LINE ( 'NONE', #7962, #9256 ) ;
#2933=DIRECTION ( 'NONE',  ( -0.000000000000000000, -0.000000000000000000, -1.000000000000000000 ) ) ;
#2939=DIRECTION ( 'NONE',  ( 1.000000000000000000, 0.000000000000000000, -0.000000000000000000 ) ) ;
#2942=EDGE_LOOP ( 'NONE', ( #9453, #368 ) ) ;
#2943=EDGE_CURVE ( 'NONE', #2819, #11286, #4048, .T. ) ;
#2944=ORIENTED_EDGE ( 'NONE', *, *, #9951, .T. ) ;
#2945=DIRECTION ( 'NONE',  ( -0.000000000000000000, -0.000000000000000000, -1.000000000000000000 ) ) ;
#2950=DIRECTION ( 'NONE',  ( -0.000000000000000000, -0.000000000000000000, -1.000000000000000000 ) ) ;
#2952=FACE_BOUND ( 'NONE', #9002, .T. ) ;
#2961=CARTESIAN_POINT ( 'NONE',  ( 50.72178482187499071, 117.2309300971526937, 3.303125000614517415 ) ) ;
#2974=CARTESIAN_POINT ( 'NONE',  ( 66.44356964374999563, 90.00000000000000000, 4.634375000614516793 ) ) ;
#2978=CIRCLE ( 'NONE', #11953, 1.500000000000001332 ) ;
#2980=CARTESIAN_POINT ( 'NONE',  ( 45.00000000000000000, 2.000000000000000000, 5.750000000000000888 ) ) ;
#2982=EDGE_CURVE ( 'NONE', #10475, #2423, #5715, .T. ) ;
#2989=VERTEX_POINT ( 'NONE', #10246 ) ;
#2993=EDGE_CURVE ( 'NONE', #2819, #6338, #2340, .T. ) ;
#2999=CARTESIAN_POINT ( 'NONE',  ( 3.800000000000015365, 90.00000000000000000, 4.212500001229034119 ) ) ;
#3007=CARTESIAN_POINT ( 'NONE',  ( 64.31840935109022439, 100.6710296186405742, 2.661976390793298286 ) ) ;
#3023=CARTESIAN_POINT ( 'NONE',  ( 35.00000000000000000, 126.0266567974326222, 3.200000001229034385 ) ) ;
#3024=( LENGTH_UNIT ( ) NAMED_UNIT ( * ) SI_UNIT ( .MILLI., .METRE. ) );
#3028=CARTESIAN_POINT ( 'NONE',  ( 19.40000000000000924, 117.0199925980744666, 3.575000000000000178 ) ) ;
#3034=CARTESIAN_POINT ( 'NONE',  ( 64.54729015011659499, 100.7543347877113717, 2.821351390178781227 ) ) ;
#3038=CARTESIAN_POINT ( 'NONE',  ( 66.44356964374998142, 108.1539533981018053, 4.615625000614516971 ) ) ;
#3044=VECTOR ( 'NONE', #3393, 1000.000000000000000 ) ;
#3046=CIRCLE ( 'NONE', #935, 1.599999999999990319 ) ;
#3049=FACE_BOUND ( 'NONE', #4853, .T. ) ;
#3055=ORIENTED_EDGE ( 'NONE', *, *, #8182, .T. ) ;
#3057=DIRECTION ( 'NONE',  ( 1.000000000000000000, 0.000000000000000000, 0.000000000000000000 ) ) ;
#3068=( BOUNDED_CURVE ( )  B_SPLINE_CURVE ( 2, ( #7082, #12055, #12316, #6232, #3103, #3169, #12254 ),
 .UNSPECIFIED., .F., .T. ) 
 B_SPLINE_CURVE_WITH_KNOTS ( ( 3, 2, 2, 3 ),
 ( 0.5000000000000001110, 0.5333333333333334370, 0.5666666666666666519, 0.5999999999999999778 ),
 .UNSPECIFIED. ) 
 CURVE ( )  GEOMETRIC_REPRESENTATION_ITEM ( )  RATIONAL_B_SPLINE_CURVE ( ( 0.9999999999999995559, 0.8660254037844391517, 1.000000000000000000, 0.8660254037844387076, 1.000000000000000000, 0.8660254037844387076, 1.000000000000000000 ) ) 
 REPRESENTATION_ITEM ( '' )  );
#3071=ORIENTED_EDGE ( 'NONE', *, *, #791, .F. ) ;
#3082=CARTESIAN_POINT ( 'NONE',  ( 35.00000000000000000, 90.00000000000000000, 5.000000000000000000 ) ) ;
#3095=ADVANCED_FACE ( 'NONE', ( #7433 ), #11550, .F. ) ;
#3098=CARTESIAN_POINT ( 'NONE',  ( 19.40000000000000924, 117.0199925980744666, 4.474999999999999645 ) ) ;
#3103=CARTESIAN_POINT ( 'NONE',  ( 19.40000000000002700, 62.98000740192551206, 3.725000000000000089 ) ) ;
#3104=ORIENTED_EDGE ( 'NONE', *, *, #11838, .F. ) ;
#3106=CARTESIAN_POINT ( 'NONE',  ( 50.72178482187499071, 117.2309300971526937, 4.653125000614517504 ) ) ;
#3108=EDGE_CURVE ( 'NONE', #5993, #4459, #10442, .T. ) ;
#3115=FACE_OUTER_BOUND ( 'NONE', #819, .T. ) ;
#3130=EDGE_CURVE ( 'NONE', #5549, #4991, #4493, .T. ) ;
#3132=DIRECTION ( 'NONE',  ( 0.000000000000000000, 0.000000000000000000, -1.000000000000000000 ) ) ;
#3141=CARTESIAN_POINT ( 'NONE',  ( 19.40000000000000924, 117.0199925980744666, 4.587500001229034119 ) ) ;
#3144=VECTOR ( 'NONE', #12283, 1000.000000000000000 ) ;
#3146=FACE_OUTER_BOUND ( 'NONE', #8120, .T. ) ;
#3159=CARTESIAN_POINT ( 'NONE',  ( 50.60000000000001563, 62.98000740192552627, 3.462500001229034563 ) ) ;
#3160=( NAMED_UNIT ( * ) SI_UNIT ( $, .STERADIAN. ) SOLID_ANGLE_UNIT ( ) );
#3164=CARTESIAN_POINT ( 'NONE',  ( 50.60000000000001563, 62.98000740192552627, 3.800000000000000266 ) ) ;
#3169=CARTESIAN_POINT ( 'NONE',  ( 3.800000000000025580, 71.98667160128366049, 3.687500000000000888 ) ) ;
#3173=CARTESIAN_POINT ( 'NONE',  ( 35.00000000000000000, 126.3079067962035822, 3.340625000614517059 ) ) ;
#3182=CARTESIAN_POINT ( 'NONE',  ( 49.99999999999996447, 90.00000000000000000, -8.000000000000000000 ) ) ;
#3186=CARTESIAN_POINT ( 'NONE',  ( 20.00000000000000355, 121.2009999999999934, 1.500000000000000444 ) ) ;
#3189=ORIENTED_EDGE ( 'NONE', *, *, #10607, .F. ) ;
#3192=DIRECTION ( 'NONE',  ( -1.000000000000000000, 0.000000000000000000, -2.891205793294679312E-17 ) ) ;
#3201=DIRECTION ( 'NONE',  ( 1.000000000000000000, 0.000000000000000000, -1.390002785237826498E-17 ) ) ;
#3203=CARTESIAN_POINT ( 'NONE',  ( 40.00000000000000000, 2.000000000000000000, 10.00000000000000000 ) ) ;
#3210=PRODUCT_DEFINITION_CONTEXT ( 'detailed design', #2088, 'design' ) ;
#3213=CARTESIAN_POINT ( 'NONE',  ( 3.800000000000015365, 90.00000000000000000, 3.762500001229034385 ) ) ;
#3217=EDGE_LOOP ( 'NONE', ( #11577, #3476, #4241, #9291, #11148, #12810, #11964, #7077 ) ) ;
#3224=CARTESIAN_POINT ( 'NONE',  ( 50.59999999999999432, 117.0199925980744666, 3.612500001229034474 ) ) ;
#3230=CARTESIAN_POINT ( 'NONE',  ( 35.00000000000000711, 53.69209320379640360, 4.521875000614516971 ) ) ;
#3236=ORIENTED_EDGE ( 'NONE', *, *, #11318, .T. ) ;
#3238=CARTESIAN_POINT ( 'NONE',  ( 50.00000000000000000, 121.2009999999999934, -1.500000000000000000 ) ) ;
#3239=CARTESIAN_POINT ( 'NONE',  ( 35.00000000000000711, 53.69209320379640360, 3.565625000614517592 ) ) ;
#3241=DIRECTION ( 'NONE',  ( 0.000000000000000000, 0.000000000000000000, -1.000000000000000000 ) ) ;
#3242=MANIFOLD_SOLID_BREP ( 'AdvancedHole1', #10097 ) ;
#3257=EDGE_LOOP ( 'NONE', ( #8053, #1252, #2350, #2230 ) ) ;
#3266=( BOUNDED_CURVE ( )  B_SPLINE_CURVE ( 2, ( #7463, #7331, #9295, #1179, #12438, #10408, #6220 ),
 .UNSPECIFIED., .F., .F. ) 
 B_SPLINE_CURVE_WITH_KNOTS ( ( 3, 2, 2, 3 ),
 ( 0.5999999999999999778, 0.6333333333333334147, 0.6666666666666667407, 0.7000000000000001776 ),
 .UNSPECIFIED. ) 
 CURVE ( )  GEOMETRIC_REPRESENTATION_ITEM ( )  RATIONAL_B_SPLINE_CURVE ( ( 1.000000000000000000, 0.8660254037844387076, 1.000000000000000000, 0.8660254037844387076, 1.000000000000000000, 0.8660254037844378194, 1.000000000000000888 ) ) 
 REPRESENTATION_ITEM ( '' )  );
#3268=CARTESIAN_POINT ( 'NONE',  ( 50.00000000000000000, 0.000000000000000000, -10.00000000000000000 ) ) ;
#3275=ADVANCED_FACE ( 'NONE', ( #2623 ), #1501, .F. ) ;
#3291=CARTESIAN_POINT ( 'NONE',  ( 50.60000000000001563, 62.98000740192552627, 4.700000000000000178 ) ) ;
#3292=CARTESIAN_POINT ( 'NONE',  ( 3.800000000000025135, 71.98667160128366049, 3.350000001229034297 ) ) ;
#3296=CARTESIAN_POINT ( 'NONE',  ( 50.60000000000001563, 62.98000740192552627, 4.250000000000000000 ) ) ;
#3302=DIRECTION ( 'NONE',  ( -0.000000000000000000, -0.000000000000000000, 1.000000000000000000 ) ) ;
#3306=CARTESIAN_POINT ( 'NONE',  ( 19.27821517812500574, 117.2309300971526937, 4.278125000614516615 ) ) ;
#3307=CARTESIAN_POINT ( 'NONE',  ( 35.00000000000000711, 53.69209320379639649, 3.621875000614517059 ) ) ;
#3314=CARTESIAN_POINT ( 'NONE',  ( 9.294992700730281499, 72.31688376601880464, -1.000000000000000000 ) ) ;
#3325=VECTOR ( 'NONE', #7351, 1000.000000000000000 ) ;
#3329=CARTESIAN_POINT ( 'NONE',  ( 45.00000000000000000, 2.000000000000001332, 7.349999999999990763 ) ) ;
#3336=EDGE_LOOP ( 'NONE', ( #5339, #10851, #11204, #8554 ) ) ;
#3339=AXIS2_PLACEMENT_3D ( 'NONE', #1913, #664, #12654 ) ;
#3345=CIRCLE ( 'NONE', #9182, 1.599999999999997202 ) ;
#3346=DIRECTION ( 'NONE',  ( -0.000000000000000000, -0.000000000000000000, -1.000000000000000000 ) ) ;
#3351=ORIENTED_EDGE ( 'NONE', *, *, #1911, .F. ) ;
#3355=CARTESIAN_POINT ( 'NONE',  ( 3.800000000000039790, 71.98667160128364628, 4.587500000000000355 ) ) ;
#3360=CARTESIAN_POINT ( 'NONE',  ( 3.556430356250028790, 71.84604660189818048, 3.546875000614516882 ) ) ;
#3365=VECTOR ( 'NONE', #11635, 1000.000000000000000 ) ;
#3373=CARTESIAN_POINT ( 'NONE',  ( 9.294992700730281499, 72.31688376601880464, 5.000000000000000000 ) ) ;
#3376=DIRECTION ( 'NONE',  ( 0.000000000000000000, 0.000000000000000000, 1.000000000000000000 ) ) ;
#3378=PLANE ( 'NONE',  #3753 ) ;
#3381=AXIS2_PLACEMENT_3D ( 'NONE', #10864, #2833, #11974 ) ;
#3385=ORIENTED_EDGE ( 'NONE', *, *, #8109, .T. ) ;
#3393=DIRECTION ( 'NONE',  ( -0.000000000000000000, -0.000000000000000000, -1.000000000000000000 ) ) ;
#3399=CARTESIAN_POINT ( 'NONE',  ( 3.800000000000135270, 108.0133283987163679, 2.825000001229033941 ) ) ;
#3400=CARTESIAN_POINT ( 'NONE',  ( 20.00000000000000355, 2.000000000000001776, -1.499999999999999556 ) ) ;
#3401=EDGE_CURVE ( 'NONE', #10264, #1821, #1954, .T. ) ;
#3402=ORIENTED_EDGE ( 'NONE', *, *, #12032, .T. ) ;
#3405=VECTOR ( 'NONE', #2945, 1000.000000000000000 ) ;
#3415=CARTESIAN_POINT ( 'NONE',  ( 35.00000000000000711, 53.97334320256736362, 4.662499999999999645 ) ) ;
#3420=CARTESIAN_POINT ( 'NONE',  ( 66.44356964374999563, 90.00000000000000000, 3.284375000614517148 ) ) ;
#3421=VERTEX_POINT ( 'NONE', #10054 ) ;
#3440=VECTOR ( 'NONE', #10110, 1000.000000000000000 ) ;
#3445=CARTESIAN_POINT ( 'NONE',  ( 20.00000000000000355, 0.000000000000000000, 10.00000000000000000 ) ) ;
#3451=EDGE_CURVE ( 'NONE', #5692, #10832, #2011, .T. ) ;
#3454=FACE_OUTER_BOUND ( 'NONE', #4254, .T. ) ;
#3463=CYLINDRICAL_SURFACE ( 'NONE', #4936, 4.999999999999997335 ) ;
#3472=FACE_OUTER_BOUND ( 'NONE', #2024, .T. ) ;
#3476=ORIENTED_EDGE ( 'NONE', *, *, #390, .F. ) ;
#3486=ORIENTED_EDGE ( 'NONE', *, *, #10138, .T. ) ;
#3490=CARTESIAN_POINT ( 'NONE',  ( 66.19999999999998863, 90.00000000000000000, 3.087500001229034119 ) ) ;
#3493=EDGE_LOOP ( 'NONE', ( #9077, #8307, #2879, #673 ) ) ;
#3499=CARTESIAN_POINT ( 'NONE',  ( 66.44356964374998142, 108.1539533981018053, 3.321875000614517237 ) ) ;
#3509=CARTESIAN_POINT ( 'NONE',  ( 66.19999999999998863, 90.00000000000000000, 4.774999999999999467 ) ) ;
#3511=VERTEX_POINT ( 'NONE', #10318 ) ;
#3518=CARTESIAN_POINT ( 'NONE',  ( 35.00000000000000000, 90.00000000000000000, 5.000000000000000000 ) ) ;
#3519=ORIENTED_EDGE ( 'NONE', *, *, #10138, .F. ) ;
#3522=CARTESIAN_POINT ( 'NONE',  ( 66.44356964375000985, 71.84604660189820891, 4.540625000614517681 ) ) ;
#3528=ORIENTED_EDGE ( 'NONE', *, *, #2794, .F. ) ;
#3537=ORIENTED_EDGE ( 'NONE', *, *, #7500, .F. ) ;
#3547=PLANE ( 'NONE',  #6006 ) ;
#3550=VECTOR ( 'NONE', #4412, 1000.000000000000000 ) ;
#3551=VERTEX_POINT ( 'NONE', #8560 ) ;
#3552=CARTESIAN_POINT ( 'NONE',  ( 3.556430356250028790, 71.84604660189818048, 3.096875000614517592 ) ) ;
#3561=FACE_OUTER_BOUND ( 'NONE', #5545, .T. ) ;
#3563=CARTESIAN_POINT ( 'NONE',  ( 66.19999999999998863, 90.00000000000000000, 3.087500001229034119 ) ) ;
#3566=CARTESIAN_POINT ( 'NONE',  ( 45.00000000000000000, 0.000000000000000000, 5.750000000000000888 ) ) ;
#3567=AXIS2_PLACEMENT_3D ( 'NONE', #3587, #1615, #8296 ) ;
#3573=CARTESIAN_POINT ( 'NONE',  ( 66.19999999999998863, 90.00000000000000000, 4.437500001229033764 ) ) ;
#3574=LINE ( 'NONE', #9581, #11628 ) ;
#3584=AXIS2_PLACEMENT_3D ( 'NONE', #8462, #2188, #4341 ) ;
#3587=CARTESIAN_POINT ( 'NONE',  ( 0.000000000000000000, 0.000000000000000000, -10.00000000000000000 ) ) ;
#3592=LINE ( 'NONE', #1745, #4331 ) ;
#3608=ORIENTED_EDGE ( 'NONE', *, *, #1382, .T. ) ;
#3618=CARTESIAN_POINT ( 'NONE',  ( 3.556430356250015024, 90.00000000000000000, 3.059375000614517059 ) ) ;
#3628=CARTESIAN_POINT ( 'NONE',  ( 66.44356964374998142, 108.1539533981018053, 4.615625000614516971 ) ) ;
#3637=CARTESIAN_POINT ( 'NONE',  ( 35.00000000000000000, 90.00000000000000000, 5.000000000000000000 ) ) ;
#3640=MECHANICAL_DESIGN_GEOMETRIC_PRESENTATION_REPRESENTATION('',(#268),#11772);
#3648=EDGE_LOOP ( 'NONE', ( #10909, #10304, #10244, #6824 ) ) ;
#3651=CARTESIAN_POINT ( 'NONE',  ( 19.27821517812500574, 117.2309300971526937, 4.278125000614516615 ) ) ;
#3653=AXIS2_PLACEMENT_3D ( 'NONE', #2329, #2266, #1134 ) ;
#3655=ORIENTED_EDGE ( 'NONE', *, *, #2223, .T. ) ;
#3661=DIRECTION ( 'NONE',  ( -0.000000000000000000, 1.000000000000000000, -0.000000000000000000 ) ) ;
#3666=VECTOR ( 'NONE', #857, 1000.000000000000000 ) ;
#3681=ORIENTED_EDGE ( 'NONE', *, *, #756, .T. ) ;
#3682=ADVANCED_FACE ( 'NONE', ( #2670 ), #3463, .F. ) ;
#3687=MECHANICAL_DESIGN_GEOMETRIC_PRESENTATION_REPRESENTATION('',(#8479),#10973);
#3688=VERTEX_POINT ( 'NONE', #9659 ) ;
#3692=DIRECTION ( 'NONE',  ( 0.000000000000000000, 0.000000000000000000, 1.000000000000000000 ) ) ;
#3693=CARTESIAN_POINT ( 'NONE',  ( 66.44356964374999563, 90.00000000000000000, 3.228125000614517237 ) ) ;
#3694=AXIS2_PLACEMENT_3D ( 'NONE', #361, #12286, #3201 ) ;
#3704=CARTESIAN_POINT ( 'NONE',  ( 35.00000000000000711, 53.69209320379640360, 3.621875000614517059 ) ) ;
#3712=EDGE_CURVE ( 'NONE', #10832, #5993, #6903, .T. ) ;
#3713=CARTESIAN_POINT ( 'NONE',  ( 35.00000000000000711, 53.69209320379639649, 3.565625000614517592 ) ) ;
#3716=EDGE_LOOP ( 'NONE', ( #4851, #7192, #157, #7403 ) ) ;
#3718=LINE ( 'NONE', #9601, #2030 ) ;
#3719=EDGE_LOOP ( 'NONE', ( #4310, #7882, #3528, #9496 ) ) ;
#3725=EDGE_LOOP ( 'NONE', ( #11303, #6580, #1876, #6450 ) ) ;
#3729=DIRECTION ( 'NONE',  ( -0.000000000000000000, -0.000000000000000000, -1.000000000000000000 ) ) ;
#3733=( NAMED_UNIT ( * ) SI_UNIT ( $, .STERADIAN. ) SOLID_ANGLE_UNIT ( ) );
#3750=CARTESIAN_POINT ( 'NONE',  ( 20.00000000000000355, 62.64236852357281293, 5.000000000000000000 ) ) ;
#3752=CARTESIAN_POINT ( 'NONE',  ( 9.294992700730283275, 72.31688376601880464, 1.000000000000000000 ) ) ;
#3753=AXIS2_PLACEMENT_3D ( 'NONE', #272, #7354, #1946 ) ;
#3754=CARTESIAN_POINT ( 'NONE',  ( 66.44356964374999563, 71.84604660189820891, 4.090625000614517504 ) ) ;
#3755=AXIS2_PLACEMENT_3D ( 'NONE', #3566, #601, #3376 ) ;
#3762=FACE_OUTER_BOUND ( 'NONE', #12367, .T. ) ;
#3764=CARTESIAN_POINT ( 'NONE',  ( 35.00000000000000000, 126.3079067962035822, 2.946875000614516793 ) ) ;
#3767=ADVANCED_FACE ( 'NONE', ( #5982 ), #7890, .T. ) ;
#3769=CARTESIAN_POINT ( 'NONE',  ( 50.59999999999999432, 117.0199925980744666, 3.612500001229034474 ) ) ;
#3776=CARTESIAN_POINT ( 'NONE',  ( 35.00000000000000000, 126.3079067962036106, 3.340625000614517504 ) ) ;
#3816=CARTESIAN_POINT ( 'NONE',  ( 66.20000000000000284, 71.98667160128370313, 3.950000001229034829 ) ) ;
#3817=ADVANCED_FACE ( 'NONE', ( #9254 ), #11147, .F. ) ;
#3825=CARTESIAN_POINT ( 'NONE',  ( 64.54728994471078352, 100.7543353520590870, 2.802601390178781404 ) ) ;
#3828=CARTESIAN_POINT ( 'NONE',  ( 19.27821517812503060, 62.76906990284727783, 4.034375000614517148 ) ) ;
#3829=ORIENTED_EDGE ( 'NONE', *, *, #1902, .T. ) ;
#3835=AXIS2_PLACEMENT_3D ( 'NONE', #4953, #5739, #4765 ) ;
#3839=CARTESIAN_POINT ( 'NONE',  ( 50.72178482187501203, 62.76906990284730625, 3.603125000614517681 ) ) ;
#3840=CARTESIAN_POINT ( 'NONE',  ( 25.00000000000000355, 2.000000000000001332, 7.349999999999986322 ) ) ;
#3842=VERTEX_POINT ( 'NONE', #1334 ) ;
#3849=PRODUCT_DEFINITION_FORMATION_WITH_SPECIFIED_SOURCE ( 'ANY', '', #1339, .NOT_KNOWN. ) ;
#3855=EDGE_LOOP ( 'NONE', ( #5618, #10401, #10940, #8946, #12770, #11323, #326, #12436, #7505, #2725, #1616, #8763 ) ) ;
#3859=CARTESIAN_POINT ( 'NONE',  ( 50.00000000000000000, 2.000000000000000000, 10.00000000000000000 ) ) ;
#3862=DIRECTION ( 'NONE',  ( -1.000000000000000000, 0.000000000000000000, 0.000000000000000000 ) ) ;
#3864=CARTESIAN_POINT ( 'NONE',  ( 20.00000000000000355, 2.000000000000001776, -1.499999999999999556 ) ) ;
#3873=EDGE_LOOP ( 'NONE', ( #4568, #3055, #189, #611 ) ) ;
#3880=AXIS2_PLACEMENT_3D ( 'NONE', #9475, #503, #4641 ) ;
#3882=CARTESIAN_POINT ( 'NONE',  ( 25.00000000000000355, 2.000000000000001332, -7.349999999999986322 ) ) ;
#3884=CARTESIAN_POINT ( 'NONE',  ( 19.27821517812503060, 62.76906990284727783, 3.078125000614517326 ) ) ;
#3889=CARTESIAN_POINT ( 'NONE',  ( 3.800000000000015365, 108.0133283987163111, 4.962499999999999467 ) ) ;
#3898=CARTESIAN_POINT ( 'NONE',  ( 50.72178482187501203, 62.76906990284730625, 3.659375000614517592 ) ) ;
#3905=FACE_OUTER_BOUND ( 'NONE', #3336, .T. ) ;
#3910=ORIENTED_EDGE ( 'NONE', *, *, #2223, .F. ) ;
#3935=VERTEX_POINT ( 'NONE', #1468 ) ;
#3945=CARTESIAN_POINT ( 'NONE',  ( 35.00000000000000000, 126.0266567974326222, 3.087499999999999911 ) ) ;
#3947=CARTESIAN_POINT ( 'NONE',  ( 35.00000000000000000, 126.3079067962035822, 4.240625000614517859 ) ) ;
#3948=CARTESIAN_POINT ( 'NONE',  ( 50.00000000000000000, 121.2009999999999934, 1.500000000000001332 ) ) ;
#3964=CARTESIAN_POINT ( 'NONE',  ( 40.00000000000000000, 90.00000000000000000, -5.000000000000000000 ) ) ;
#3966=VECTOR ( 'NONE', #9497, 1000.000000000000000 ) ;
#3973=ORIENTED_EDGE ( 'NONE', *, *, #4201, .F. ) ;
#3978=DIRECTION ( 'NONE',  ( 0.000000000000000000, 1.000000000000000000, 0.000000000000000000 ) ) ;
#3979=CARTESIAN_POINT ( 'NONE',  ( 50.59999999999999432, 117.0199925980744666, 3.500000000000000444 ) ) ;
#3981=DIRECTION ( 'NONE',  ( -0.000000000000000000, 1.000000000000000000, -0.000000000000000000 ) ) ;
#3997=ORIENTED_EDGE ( 'NONE', *, *, #4300, .T. ) ;
#3999=ORIENTED_EDGE ( 'NONE', *, *, #1331, .F. ) ;
#4002=EDGE_CURVE ( 'NONE', #10475, #8376, #3574, .T. ) ;
#4005=FACE_OUTER_BOUND ( 'NONE', #8761, .T. ) ;
#4007=DIRECTION ( 'NONE',  ( -1.000000000000000000, -0.000000000000000000, -0.000000000000000000 ) ) ;
#4009=DIRECTION ( 'NONE',  ( -0.000000000000000000, -0.000000000000000000, -1.000000000000000000 ) ) ;
#4010=CARTESIAN_POINT ( 'NONE',  ( 3.800000000000015365, 90.00000000000000000, 2.862500001229034474 ) ) ;
#4015=ORIENTED_EDGE ( 'NONE', *, *, #4317, .F. ) ;
#4016=LINE ( 'NONE', #4799, #3666 ) ;
#4020=DIRECTION ( 'NONE',  ( -0.000000000000000000, -0.000000000000000000, -1.000000000000000000 ) ) ;
#4023=CARTESIAN_POINT ( 'NONE',  ( 66.44356964374999563, 90.00000000000000000, 4.578125000614516438 ) ) ;
#4034=ADVANCED_FACE ( 'NONE', ( #4678 ), #2149, .F. ) ;
#4040=FACE_OUTER_BOUND ( 'NONE', #3217, .T. ) ;
#4041=CARTESIAN_POINT ( 'NONE',  ( 20.00000000000000355, 0.000000000000000000, 10.00000000000000000 ) ) ;
#4048=CIRCLE ( 'NONE', #4457, 1.599999999999997202 ) ;
#4053=VERTEX_POINT ( 'NONE', #7150 ) ;
#4054=CARTESIAN_POINT ( 'NONE',  ( 3.800000000000015365, 90.00000000000000000, 4.100000000000000533 ) ) ;
#4055=CARTESIAN_POINT ( 'NONE',  ( 35.00000000000000000, 90.00000000000000000, -5.000000000000000000 ) ) ;
#4059=DIRECTION ( 'NONE',  ( 0.000000000000000000, 0.000000000000000000, 1.000000000000000000 ) ) ;
#4073=CARTESIAN_POINT ( 'NONE',  ( 3.800000000000015365, 108.0133283987163111, 2.825000001229034385 ) ) ;
#4077=CARTESIAN_POINT ( 'NONE',  ( 19.40000000000002700, 62.98000740192551206, 3.725000000000000089 ) ) ;
#4086=CARTESIAN_POINT ( 'NONE',  ( 50.72178482187501203, 62.76906990284730625, 3.153125000614517504 ) ) ;
#4105=CARTESIAN_POINT ( 'NONE',  ( 66.19999999999998863, 90.00000000000000000, 3.425000000000000266 ) ) ;
#4106=CARTESIAN_POINT ( 'NONE',  ( 35.00000000000000000, 90.00000000000000000, 5.000000000000000000 ) ) ;
#4107=ADVANCED_FACE ( 'NONE', ( #3561 ), #9435, .F. ) ;
#4109=ORIENTED_EDGE ( 'NONE', *, *, #5242, .T. ) ;
#4112=ORIENTED_EDGE ( 'NONE', *, *, #11318, .F. ) ;
#4124=EDGE_LOOP ( 'NONE', ( #3351, #6950, #8065, #5022 ) ) ;
#4126=PLANE ( 'NONE',  #11392 ) ;
#4138=CARTESIAN_POINT ( 'NONE',  ( 66.19999999999997442, 108.0133283987163253, 3.125000001229034208 ) ) ;
#4140=CARTESIAN_POINT ( 'NONE',  ( 12.66025403784434822, 85.80682368868758658, -1.000000000000000000 ) ) ;
#4142=CARTESIAN_POINT ( 'NONE',  ( 19.40000000000002700, 62.98000740192551206, 4.174999999999999822 ) ) ;
#4147=DIRECTION ( 'NONE',  ( -0.000000000000000000, 1.000000000000000000, -0.000000000000000000 ) ) ;
#4158=DIRECTION ( 'NONE',  ( 0.000000000000000000, -1.000000000000000000, 0.000000000000000000 ) ) ;
#4190=DIRECTION ( 'NONE',  ( -1.000000000000000000, 0.000000000000000000, -0.000000000000000000 ) ) ;
#4192=PRODUCT_CONTEXT ( 'NONE', #11522, 'mechanical' ) ;
#4195=LINE ( 'NONE', #9026, #6963 ) ;
#4201=EDGE_CURVE ( 'NONE', #10118, #2032, #760, .T. ) ;
#4207=CARTESIAN_POINT ( 'NONE',  ( 50.59999999999999432, 117.0199925980744666, 3.950000000000000178 ) ) ;
#4211=LINE ( 'NONE', #1189, #892 ) ;
#4216=CARTESIAN_POINT ( 'NONE',  ( 35.00000000000000000, 126.3079067962035822, 3.790625000614517237 ) ) ;
#4218=VERTEX_POINT ( 'NONE', #6617 ) ;
#4219=PLANE ( 'NONE',  #6313 ) ;
#4222=CARTESIAN_POINT ( 'NONE',  ( 35.00000000000000000, 90.00000000000000000, 5.000000000000000000 ) ) ;
#4235=CIRCLE ( 'NONE', #2563, 1.599999999999986766 ) ;
#4236=EDGE_CURVE ( 'NONE', #4511, #10380, #770, .T. ) ;
#4241=ORIENTED_EDGE ( 'NONE', *, *, #2794, .T. ) ;
#4251=VERTEX_POINT ( 'NONE', #10617 ) ;
#4254=EDGE_LOOP ( 'NONE', ( #7776, #8432, #10122, #3910 ) ) ;
#4260=ORIENTED_EDGE ( 'NONE', *, *, #3451, .T. ) ;
#4266=CARTESIAN_POINT ( 'NONE',  ( 19.40000000000000924, 117.0199925980744666, 3.687500001229034208 ) ) ;
#4271=CARTESIAN_POINT ( 'NONE',  ( 19.27821517812503060, 62.76906990284727783, 4.484375000614516438 ) ) ;
#4276=VECTOR ( 'NONE', #8277, 1000.000000000000000 ) ;
#4277=CARTESIAN_POINT ( 'NONE',  ( 30.00000000000000711, 90.00000000000000000, -10.00000000000000000 ) ) ;
#4278=VERTEX_POINT ( 'NONE', #3882 ) ;
#4281=CARTESIAN_POINT ( 'NONE',  ( 19.27821517812500574, 117.2309300971526937, 2.928125000614517415 ) ) ;
#4282=CARTESIAN_POINT ( 'NONE',  ( 3.556430356250028790, 71.84604660189818048, 3.546875000614517326 ) ) ;
#4294=AXIS2_PLACEMENT_3D ( 'NONE', #4431, #6385, #11162 ) ;
#4300=EDGE_CURVE ( 'NONE', #1050, #4594, #7914, .T. ) ;
#4302=DIRECTION ( 'NONE',  ( 1.000000000000000000, 0.000000000000000000, 0.000000000000000000 ) ) ;
#4307=CARTESIAN_POINT ( 'NONE',  ( 22.99999999999998579, 90.00000000000000000, -8.000000000000000000 ) ) ;
#4310=ORIENTED_EDGE ( 'NONE', *, *, #8400, .T. ) ;
#4314=CARTESIAN_POINT ( 'NONE',  ( 60.43447243729646345, 111.3420572890633764, 2.688859442485532991 ) ) ;
#4317=EDGE_CURVE ( 'NONE', #5941, #10632, #8655, .T. ) ;
#4320=ORIENTED_EDGE ( 'NONE', *, *, #8258, .T. ) ;
#4331=VECTOR ( 'NONE', #7445, 1000.000000000000000 ) ;
#4334=CARTESIAN_POINT ( 'NONE',  ( 3.800000000000015365, 90.00000000000000000, 4.549999999999999822 ) ) ;
#4339=ORIENTED_EDGE ( 'NONE', *, *, #1699, .T. ) ;
#4340=CIRCLE ( 'NONE', #8308, 1.599999999999986766 ) ;
#4341=DIRECTION ( 'NONE',  ( 1.000000000000000000, 0.000000000000000000, 0.000000000000000000 ) ) ;
#4343=CARTESIAN_POINT ( 'NONE',  ( 66.44356964375000985, 71.84604660189820891, 3.246875000614517504 ) ) ;
#4347=DIRECTION ( 'NONE',  ( -1.000000000000000000, 0.000000000000000000, 0.000000000000000000 ) ) ;
#4349=FACE_OUTER_BOUND ( 'NONE', #2942, .T. ) ;
#4350=LINE ( 'NONE', #6914, #11472 ) ;
#4358=AXIS2_PLACEMENT_3D ( 'NONE', #4055, #2027, #1960 ) ;
#4360=EDGE_LOOP ( 'NONE', ( #6330, #18, #11832, #4452 ) ) ;
#4364=CARTESIAN_POINT ( 'NONE',  ( 45.00000000000000000, 2.000000000000000000, -4.150000000000005684 ) ) ;
#4369=CARTESIAN_POINT ( 'NONE',  ( 3.556430356250014579, 108.1539533981018053, 4.765625000614517326 ) ) ;
#4372=ORIENTED_EDGE ( 'NONE', *, *, #2781, .F. ) ;
#4386=CARTESIAN_POINT ( 'NONE',  ( 66.19999999999988916, 71.98667160128361786, 3.387499999999999734 ) ) ;
#4389=ORIENTED_EDGE ( 'NONE', *, *, #9963, .T. ) ;
#4396=VERTEX_POINT ( 'NONE', #5671 ) ;
#4397=ADVANCED_FACE ( 'NONE', ( #11428, #10452 ), #4569, .F. ) ;
#4398=CARTESIAN_POINT ( 'NONE',  ( 50.72178482187501203, 62.76906990284730625, 4.109375000614517326 ) ) ;
#4409=CARTESIAN_POINT ( 'NONE',  ( 5.011331584521383498, 81.39071625125095011, 1.000000000000000000 ) ) ;
#4412=DIRECTION ( 'NONE',  ( -0.000000000000000000, -0.000000000000000000, -1.000000000000000000 ) ) ;
#4413=EDGE_CURVE ( 'NONE', #10818, #7686, #3718, .T. ) ;
#4419=CARTESIAN_POINT ( 'NONE',  ( 45.00000000000000000, 2.000000000000001332, 4.150000000000010125 ) ) ;
#4431=CARTESIAN_POINT ( 'NONE',  ( 35.00000000000000000, 90.00000000000000000, -8.000000000000000000 ) ) ;
#4449=ADVANCED_FACE ( 'NONE', ( #11493 ), #9724, .T. ) ;
#4450=VERTEX_POINT ( 'NONE', #7509 ) ;
#4451=( LENGTH_UNIT ( ) NAMED_UNIT ( * ) SI_UNIT ( .MILLI., .METRE. ) );
#4452=ORIENTED_EDGE ( 'NONE', *, *, #11511, .T. ) ;
#4456=DIRECTION ( 'NONE',  ( -0.000000000000000000, 1.000000000000000000, -0.000000000000000000 ) ) ;
#4457=AXIS2_PLACEMENT_3D ( 'NONE', #7107, #9066, #2278 ) ;
#4459=VERTEX_POINT ( 'NONE', #1685 ) ;
#4466=DIRECTION ( 'NONE',  ( 1.000000000000000000, 0.000000000000000000, -0.000000000000000000 ) ) ;
#4467=VECTOR ( 'NONE', #12474, 1000.000000000000000 ) ;
#4469=CARTESIAN_POINT ( 'NONE',  ( 19.27821517812503060, 62.76906990284727783, 3.584375000614516971 ) ) ;
#4470=CARTESIAN_POINT ( 'NONE',  ( 66.44356964374999563, 71.84604660189820891, 4.540625000614517681 ) ) ;
#4475=VECTOR ( 'NONE', #5260, 1000.000000000000000 ) ;
#4477=FACE_OUTER_BOUND ( 'NONE', #12786, .T. ) ;
#4485=LINE ( 'NONE', #3203, #4647 ) ;
#4493=LINE ( 'NONE', #1539, #316 ) ;
#4494=CYLINDRICAL_SURFACE ( 'NONE', #9069, 31.19999999999998863 ) ;
#4498=CARTESIAN_POINT ( 'NONE',  ( 50.72178482187501203, 62.76906990284730625, 4.503125000614517148 ) ) ;
#4503=DIRECTION ( 'NONE',  ( -1.000000000000000000, 0.000000000000000000, 0.000000000000000000 ) ) ;
#4508=EDGE_CURVE ( 'NONE', #6922, #6195, #3592, .T. ) ;
#4511=VERTEX_POINT ( 'NONE', #7573 ) ;
#4523=ORIENTED_EDGE ( 'NONE', *, *, #9782, .F. ) ;
#4529=CARTESIAN_POINT ( 'NONE',  ( 66.44356964374998142, 108.1539533981018053, 3.771875000614516971 ) ) ;
#4539=CARTESIAN_POINT ( 'NONE',  ( 3.556430356250015024, 90.00000000000000000, 4.803125000614516971 ) ) ;
#4540=CARTESIAN_POINT ( 'NONE',  ( 25.00000000000000355, 2.000000000000000000, 5.750000000000000000 ) ) ;
#4561=DIRECTION ( 'NONE',  ( -0.000000000000000000, -0.000000000000000000, -1.000000000000000000 ) ) ;
#4568=ORIENTED_EDGE ( 'NONE', *, *, #791, .T. ) ;
#4569=PLANE ( 'NONE',  #1610 ) ;
#4571=CARTESIAN_POINT ( 'NONE',  ( 30.00000000000000711, 90.00000000000000000, -5.000000000000000000 ) ) ;
#4574=AXIS2_PLACEMENT_3D ( 'NONE', #5222, #10001, #10060 ) ;
#4592=CARTESIAN_POINT ( 'NONE',  ( 35.00000000000000711, 53.69209320379640360, 3.171875000614517326 ) ) ;
#4594=VERTEX_POINT ( 'NONE', #6969 ) ;
#4602=CARTESIAN_POINT ( 'NONE',  ( 40.00000000000000000, 121.2009999999999934, 1.500000000000001110 ) ) ;
#4605=CARTESIAN_POINT ( 'NONE',  ( 3.800000000000015365, 90.00000000000000000, 3.312500001229034652 ) ) ;
#4606=FACE_OUTER_BOUND ( 'NONE', #3725, .T. ) ;
#4610=ADVANCED_FACE ( 'NONE', ( #11752, #9790, #6779, #10771 ), #6906, .F. ) ;
#4623=ADVANCED_FACE ( 'NONE', ( #5984 ), #4822, .F. ) ;
#4625=VECTOR ( 'NONE', #9173, 1000.000000000000000 ) ;
#4628=CARTESIAN_POINT ( 'NONE',  ( 3.556430356250015024, 90.00000000000000000, 4.353125000614517681 ) ) ;
#4637=VECTOR ( 'NONE', #658, 1000.000000000000000 ) ;
#4641=DIRECTION ( 'NONE',  ( -1.000000000000000000, 0.000000000000000000, 0.000000000000000000 ) ) ;
#4647=VECTOR ( 'NONE', #9387, 1000.000000000000000 ) ;
#4655=UNCERTAINTY_MEASURE_WITH_UNIT (LENGTH_MEASURE( 1.000000000000000082E-05 ), #3024, 'distance_accuracy_value', 'NONE');
#4658=CARTESIAN_POINT ( 'NONE',  ( 19.27821517812503060, 62.76906990284727783, 3.584375000614516971 ) ) ;
#4663=ORIENTED_EDGE ( 'NONE', *, *, #2733, .T. ) ;
#4675=VECTOR ( 'NONE', #10712, 1000.000000000000227 ) ;
#4678=FACE_OUTER_BOUND ( 'NONE', #2890, .T. ) ;
#4693=CARTESIAN_POINT ( 'NONE',  ( 66.44356964374999563, 90.00000000000000000, 3.678125000614516971 ) ) ;
#4699=ORIENTED_EDGE ( 'NONE', *, *, #8839, .F. ) ;
#4705=AXIS2_PLACEMENT_3D ( 'NONE', #9049, #11211, #1267 ) ;
#4721=EDGE_LOOP ( 'NONE', ( #1992, #8667, #7049, #12501, #6935 ) ) ;
#4724=DIRECTION ( 'NONE',  ( 0.000000000000000000, -1.000000000000000000, 0.000000000000000000 ) ) ;
#4732=CARTESIAN_POINT ( 'NONE',  ( 50.60000000000001563, 62.98000740192552627, 4.362500001229034474 ) ) ;
#4738=CARTESIAN_POINT ( 'NONE',  ( 64.54729015011659499, 100.7543347877113717, 2.840101390178781049 ) ) ;
#4741=CARTESIAN_POINT ( 'NONE',  ( 3.556430356250015024, 90.00000000000000000, 3.059375000614517059 ) ) ;
#4746=EDGE_LOOP ( 'NONE', ( #6394, #7273, #2614, #5268 ) ) ;
#4765=DIRECTION ( 'NONE',  ( -1.000000000000000000, 0.000000000000000000, 0.000000000000000000 ) ) ;
#4771=DIRECTION ( 'NONE',  ( -0.000000000000000000, 1.000000000000000000, -0.000000000000000000 ) ) ;
#4789=DIRECTION ( 'NONE',  ( 0.000000000000000000, 0.000000000000000000, 1.000000000000000000 ) ) ;
#4793=CARTESIAN_POINT ( 'NONE',  ( 19.27821517812500574, 117.2309300971526937, 3.378125000614517148 ) ) ;
#4799=CARTESIAN_POINT ( 'NONE',  ( 66.19999999999998863, 90.00000000000000000, 5.000000000000000000 ) ) ;
#4806=CARTESIAN_POINT ( 'NONE',  ( 64.54728994471078352, 100.7543353520590870, 2.858851390178780871 ) ) ;
#4813=DIRECTION ( 'NONE',  ( -0.000000000000000000, 1.000000000000000000, -0.000000000000000000 ) ) ;
#4814=DIRECTION ( 'NONE',  ( -0.000000000000000000, 1.000000000000000000, -0.000000000000000000 ) ) ;
#4816=CARTESIAN_POINT ( 'NONE',  ( 19.27821517812503060, 62.76906990284727783, 3.528125000614517059 ) ) ;
#4822=PLANE ( 'NONE',  #11640 ) ;
#4824=DIRECTION ( 'NONE',  ( 0.000000000000000000, 0.000000000000000000, 1.000000000000000000 ) ) ;
#4828=DIRECTION ( 'NONE',  ( 1.000000000000000000, 0.000000000000000000, 0.000000000000000000 ) ) ;
#4838=VECTOR ( 'NONE', #4007, 1000.000000000000000 ) ;
#4851=ORIENTED_EDGE ( 'NONE', *, *, #1699, .F. ) ;
#4853=EDGE_LOOP ( 'NONE', ( #5228, #2671, #280, #8620 ) ) ;
#4855=DIRECTION ( 'NONE',  ( -0.000000000000000000, 1.000000000000000000, -0.000000000000000000 ) ) ;
#4857=CARTESIAN_POINT ( 'NONE',  ( 3.800000000000015365, 108.0133283987163111, 4.175000001229034474 ) ) ;
#4861=CARTESIAN_POINT ( 'NONE',  ( 50.00000000000000000, 2.000000000000000000, 10.00000000000000000 ) ) ;
#4863=CARTESIAN_POINT ( 'NONE',  ( 3.800000000000015365, 90.00000000000000000, 3.200000000000000178 ) ) ;
#4867=CARTESIAN_POINT ( 'NONE',  ( 35.00000000000000000, 126.3079067962035822, 3.846875000614517592 ) ) ;
#4870=CYLINDRICAL_SURFACE ( 'NONE', #1201, 1.599999999999993872 ) ;
#4876=CARTESIAN_POINT ( 'NONE',  ( 35.00000000000000000, 90.00000000000000000, 5.000000000000000000 ) ) ;
#4877=DIRECTION ( 'NONE',  ( -0.8660254037844365982, -0.5000000000000036637, 0.000000000000000000 ) ) ;
#4886=DIRECTION ( 'NONE',  ( 1.000000000000000000, 0.000000000000000000, 0.000000000000000000 ) ) ;
#4896=DIRECTION ( 'NONE',  ( 1.000000000000000000, 0.000000000000000000, 0.000000000000000000 ) ) ;
#4907=ORIENTED_EDGE ( 'NONE', *, *, #12433, .F. ) ;
#4910=DIRECTION ( 'NONE',  ( 1.000000000000000000, 0.000000000000000000, 0.000000000000000000 ) ) ;
#4912=EDGE_CURVE ( 'NONE', #4450, #12839, #5593, .T. ) ;
#4915=VERTEX_POINT ( 'NONE', #12468 ) ;
#4917=CARTESIAN_POINT ( 'NONE',  ( 3.800000000000135270, 108.0133283987163679, 3.162500000000000533 ) ) ;
#4920=CARTESIAN_POINT ( 'NONE',  ( 3.556430356250028790, 71.84604660189818048, 3.940625000614518036 ) ) ;
#4929=ORIENTED_EDGE ( 'NONE', *, *, #4236, .T. ) ;
#4934=CARTESIAN_POINT ( 'NONE',  ( 3.556430356250014579, 108.1539533981018053, 3.921875000614517326 ) ) ;
#4936=AXIS2_PLACEMENT_3D ( 'NONE', #1683, #12481, #5669 ) ;
#4942=DIRECTION ( 'NONE',  ( 0.000000000000000000, 0.000000000000000000, 1.000000000000000000 ) ) ;
#4953=CARTESIAN_POINT ( 'NONE',  ( 35.00000000000000000, 90.00000000000000000, -8.000000000000000000 ) ) ;
#4955=ORIENTED_EDGE ( 'NONE', *, *, #2926, .T. ) ;
#4965=CARTESIAN_POINT ( 'NONE',  ( 64.39470308771990403, 100.6987976320522336, 2.708851390588459029 ) ) ;
#4975=AXIS2_PLACEMENT_3D ( 'NONE', #12803, #5804, #9795 ) ;
#4976=ORIENTED_EDGE ( 'NONE', *, *, #4986, .F. ) ;
#4980=CARTESIAN_POINT ( 'NONE',  ( 19.40000000000002700, 62.98000740192551206, 3.387500001229033941 ) ) ;
#4985=CARTESIAN_POINT ( 'NONE',  ( 50.59999999999999432, 117.0199925980744666, 4.850000000000000533 ) ) ;
#4986=EDGE_CURVE ( 'NONE', #5993, #8371, #11994, .T. ) ;
#4991=VERTEX_POINT ( 'NONE', #3964 ) ;
#4995=CARTESIAN_POINT ( 'NONE',  ( 66.44356964374999563, 90.00000000000000000, 4.128125000614517148 ) ) ;
#5000=AXIS2_PLACEMENT_3D ( 'NONE', #905, #7855, #4910 ) ;
#5003=CYLINDRICAL_SURFACE ( 'NONE', #2184, 30.19999999999998863 ) ;
#5011=EDGE_CURVE ( 'NONE', #7582, #11451, #5798, .T. ) ;
#5012=CARTESIAN_POINT ( 'NONE',  ( 35.00000000000000000, 126.0266567974326222, 3.537499999999999645 ) ) ;
#5013=CARTESIAN_POINT ( 'NONE',  ( 40.00000000000000000, 2.000000000000000000, 10.00000000000000000 ) ) ;
#5022=ORIENTED_EDGE ( 'NONE', *, *, #301, .F. ) ;
#5028=CARTESIAN_POINT ( 'NONE',  ( 30.00000000000000711, 0.000000000000000000, 1.500000000000000666 ) ) ;
#5036=CYLINDRICAL_SURFACE ( 'NONE', #10927, 1.599999999999992095 ) ;
#5037=EDGE_CURVE ( 'NONE', #10351, #2190, #4340, .T. ) ;
#5039=EDGE_CURVE ( 'NONE', #8420, #193, #6073, .T. ) ;
#5045=CARTESIAN_POINT ( 'NONE',  ( 3.800000000000015365, 108.0133283987163111, 3.162500000000000533 ) ) ;
#5047=CARTESIAN_POINT ( 'NONE',  ( 45.00000000000000000, 2.000000000000001332, -7.349999999999989875 ) ) ;
#5060=PLANE ( 'NONE',  #4705 ) ;
#5070=ADVANCED_FACE ( 'NONE', ( #1865 ), #4870, .F. ) ;
#5078=CARTESIAN_POINT ( 'NONE',  ( 3.800000000000001155, 108.0133283987163111, 4.175000001229035362 ) ) ;
#5079=EDGE_LOOP ( 'NONE', ( #2395, #3486, #7111, #2465 ) ) ;
#5097=PLANE ( 'NONE',  #5495 ) ;
#5104=CARTESIAN_POINT ( 'NONE',  ( 66.19999999999997442, 108.0133283987163253, 3.575000001229033941 ) ) ;
#5105=DIRECTION ( 'NONE',  ( 0.000000000000000000, 0.000000000000000000, 1.000000000000000000 ) ) ;
#5108=EDGE_CURVE ( 'NONE', #9462, #5352, #8078, .T. ) ;
#5109=CARTESIAN_POINT ( 'NONE',  ( 3.556430356250014579, 108.1539533981018053, 4.821875000614516793 ) ) ;
#5119=CARTESIAN_POINT ( 'NONE',  ( 3.556430356250015024, 90.00000000000000000, 3.453125000614517770 ) ) ;
#5128=CARTESIAN_POINT ( 'NONE',  ( 45.00000000000000000, 0.000000000000000000, 4.150000000000003908 ) ) ;
#5143=EDGE_LOOP ( 'NONE', ( #10082, #1369, #5181, #1354 ) ) ;
#5160=ORIENTED_EDGE ( 'NONE', *, *, #5039, .T. ) ;
#5173=( NAMED_UNIT ( * ) PLANE_ANGLE_UNIT ( ) SI_UNIT ( $, .RADIAN. ) );
#5177=CARTESIAN_POINT ( 'NONE',  ( 3.800000000000025135, 71.98667160128366049, 3.687500000000000888 ) ) ;
#5181=ORIENTED_EDGE ( 'NONE', *, *, #10833, .T. ) ;
#5186=CARTESIAN_POINT ( 'NONE',  ( 19.27821517812503060, 62.76906990284727783, 4.428125000614516971 ) ) ;
#5193=CARTESIAN_POINT ( 'NONE',  ( 66.19999999999998863, 90.00000000000000000, 3.987500001229034030 ) ) ;
#5196=CARTESIAN_POINT ( 'NONE',  ( 66.19999999999998863, 90.00000000000000000, 5.000000000000000000 ) ) ;
#5197=CARTESIAN_POINT ( 'NONE',  ( 49.99999999999996447, 90.00000000000000000, -8.000000000000000000 ) ) ;
#5210=CARTESIAN_POINT ( 'NONE',  ( 30.00000000000000711, 0.000000000000000000, 10.00000000000000000 ) ) ;
#5219=LINE ( 'NONE', #2153, #6304 ) ;
#5222=CARTESIAN_POINT ( 'NONE',  ( 25.00000000000000355, 2.000000000000000000, 5.750000000000000000 ) ) ;
#5227=DIRECTION ( 'NONE',  ( -0.000000000000000000, 1.000000000000000000, -0.000000000000000000 ) ) ;
#5228=ORIENTED_EDGE ( 'NONE', *, *, #4508, .F. ) ;
#5229=SHAPE_DEFINITION_REPRESENTATION ( #12317, #11692 ) ;
#5242=EDGE_CURVE ( 'NONE', #3935, #5315, #11271, .T. ) ;
#5246=CARTESIAN_POINT ( 'NONE',  ( 3.800000000000015365, 108.0133283987163111, 4.062500000000000000 ) ) ;
#5251=VERTEX_POINT ( 'NONE', #5578 ) ;
#5253=CARTESIAN_POINT ( 'NONE',  ( 19.27821517812503060, 62.76906990284727783, 3.078125000614517326 ) ) ;
#5255=CARTESIAN_POINT ( 'NONE',  ( 3.556430356250014579, 108.1539533981018053, 4.371875000614516615 ) ) ;
#5260=DIRECTION ( 'NONE',  ( 0.000000000000000000, 1.000000000000000000, 0.000000000000000000 ) ) ;
#5268=ORIENTED_EDGE ( 'NONE', *, *, #5678, .F. ) ;
#5275=VERTEX_POINT ( 'NONE', #4605 ) ;
#5278=ORIENTED_EDGE ( 'NONE', *, *, #11181, .T. ) ;
#5282=VERTEX_POINT ( 'NONE', #3563 ) ;
#5292=VECTOR ( 'NONE', #2933, 1000.000000000000000 ) ;
#5307=CARTESIAN_POINT ( 'NONE',  ( 19.40000000000002700, 62.98000740192551206, 4.625000000000000000 ) ) ;
#5311=VECTOR ( 'NONE', #12266, 1000.000000000000000 ) ;
#5312=DIRECTION ( 'NONE',  ( -1.000000000000000000, 0.000000000000000000, 0.000000000000000000 ) ) ;
#5315=VERTEX_POINT ( 'NONE', #461 ) ;
#5317=DIRECTION ( 'NONE',  ( -1.000000000000000000, 0.000000000000000000, 0.000000000000000000 ) ) ;
#5330=VECTOR ( 'NONE', #12492, 1000.000000000000000 ) ;
#5335=VECTOR ( 'NONE', #4877, 1000.000000000000000 ) ;
#5339=ORIENTED_EDGE ( 'NONE', *, *, #6683, .F. ) ;
#5352=VERTEX_POINT ( 'NONE', #4409 ) ;
#5359=CARTESIAN_POINT ( 'NONE',  ( 25.00000000000000355, 2.000000000000000000, 4.150000000000007461 ) ) ;
#5362=ADVANCED_FACE ( 'NONE', ( #5645 ), #6148, .F. ) ;
#5368=CARTESIAN_POINT ( 'NONE',  ( 3.556430356250014579, 108.1539533981018053, 3.021875000614517415 ) ) ;
#5370=CARTESIAN_POINT ( 'NONE',  ( 50.00000000000000000, 2.000000000000000000, 10.00000000000000000 ) ) ;
#5379=CARTESIAN_POINT ( 'NONE',  ( 3.800000000000015365, 90.00000000000000000, 5.000000000000000000 ) ) ;
#5384=CYLINDRICAL_SURFACE ( 'NONE', #8033, 1.500000000000001332 ) ;
#5395=CARTESIAN_POINT ( 'NONE',  ( 40.00000000000000000, 121.2009999999999934, -1.499999999999999778 ) ) ;
#5410=CARTESIAN_POINT ( 'NONE',  ( 20.00000000000000355, 0.000000000000000000, -10.00000000000000000 ) ) ;
#5435=DIRECTION ( 'NONE',  ( -1.000000000000000000, 0.000000000000000000, 0.000000000000000000 ) ) ;
#5443=CARTESIAN_POINT ( 'NONE',  ( 19.27821517812503060, 62.76906990284727783, 4.034375000614517148 ) ) ;
#5448=CARTESIAN_POINT ( 'NONE',  ( 19.40000000000002700, 62.98000740192551206, 3.837500001229034563 ) ) ;
#5449=DIRECTION ( 'NONE',  ( 0.000000000000000000, 0.000000000000000000, 1.000000000000000000 ) ) ;
#5464=EDGE_CURVE ( 'NONE', #9108, #767, #10615, .T. ) ;
#5466=LINE ( 'NONE', #11422, #3144 ) ;
#5471=ORIENTED_EDGE ( 'NONE', *, *, #10260, .F. ) ;
#5480=CYLINDRICAL_SURFACE ( 'NONE', #3880, 31.19999999999998863 ) ;
#5484=CARTESIAN_POINT ( 'NONE',  ( 35.00000000000000711, 53.97334320256736362, 3.312500000000000000 ) ) ;
#5488=ORIENTED_EDGE ( 'NONE', *, *, #6703, .T. ) ;
#5494=B_SPLINE_CURVE_WITH_KNOTS ( 'NONE', 3,
 ( #3007, #4965, #12226, #2092 ),
 .UNSPECIFIED., .F., .F.,
 ( 4, 4 ),
 ( 0.000000000000000000, 1.000000000000000000 ),
 .UNSPECIFIED. ) ;
#5495=AXIS2_PLACEMENT_3D ( 'NONE', #11971, #7003, #46 ) ;
#5497=CARTESIAN_POINT ( 'NONE',  ( 35.00000000000000000, 126.3079067962035822, 3.396875000614517415 ) ) ;
#5506=LINE ( 'NONE', #3750, #1062 ) ;
#5509=CARTESIAN_POINT ( 'NONE',  ( 35.00000000000000000, 126.3079067962036106, 2.946875000614516793 ) ) ;
#5510=CARTESIAN_POINT ( 'NONE',  ( 3.556430356250015024, 90.00000000000000000, 4.353125000614517681 ) ) ;
#5535=LINE ( 'NONE', #4307, #12327 ) ;
#5545=EDGE_LOOP ( 'NONE', ( #2093, #4389, #12867, #3999 ) ) ;
#5549=VERTEX_POINT ( 'NONE', #9296 ) ;
#5551=ORIENTED_EDGE ( 'NONE', *, *, #12947, .F. ) ;
#5558=ORIENTED_EDGE ( 'NONE', *, *, #5856, .T. ) ;
#5562=CARTESIAN_POINT ( 'NONE',  ( 50.60000000000001563, 62.98000740192552627, 4.250000000000000000 ) ) ;
#5568=CARTESIAN_POINT ( 'NONE',  ( 35.00000000000000000, 126.3079067962035822, 3.846875000614517592 ) ) ;
#5570=CARTESIAN_POINT ( 'NONE',  ( 20.00000000000000355, 2.000000000000000000, -10.00000000000000000 ) ) ;
#5576=AXIS2_PLACEMENT_3D ( 'NONE', #2608, #8563, #4503 ) ;
#5578=CARTESIAN_POINT ( 'NONE',  ( 40.00000000000000000, 2.000000000000001776, 1.500000000000001110 ) ) ;
#5581=CARTESIAN_POINT ( 'NONE',  ( 50.00000000000000000, 2.000000000000000000, 10.00000000000000000 ) ) ;
#5593=LINE ( 'NONE', #8669, #11222 ) ;
#5597=CARTESIAN_POINT ( 'NONE',  ( 3.556430356250015024, 90.00000000000000000, 4.831250000614517148 ) ) ;
#5604=CIRCLE ( 'NONE', #4358, 30.19999999999999218 ) ;
#5605=ADVANCED_FACE ( 'NONE', ( #6478 ), #3547, .F. ) ;
#5610=DIRECTION ( 'NONE',  ( 0.000000000000000000, -0.000000000000000000, -1.000000000000000000 ) ) ;
#5618=ORIENTED_EDGE ( 'NONE', *, *, #10898, .F. ) ;
#5633=ORIENTED_EDGE ( 'NONE', *, *, #4236, .F. ) ;
#5634=CARTESIAN_POINT ( 'NONE',  ( 19.27821517812503060, 62.76906990284727783, 4.034375000614517148 ) ) ;
#5635=EDGE_LOOP ( 'NONE', ( #9481, #10770 ) ) ;
#5642=CARTESIAN_POINT ( 'NONE',  ( 64.31840976852106451, 100.6710284717588166, 2.999476386674974737 ) ) ;
#5645=FACE_OUTER_BOUND ( 'NONE', #3855, .T. ) ;
#5648=DIRECTION ( 'NONE',  ( 0.000000000000000000, 0.000000000000000000, 1.000000000000000000 ) ) ;
#5655=ORIENTED_EDGE ( 'NONE', *, *, #5037, .F. ) ;
#5666=CARTESIAN_POINT ( 'NONE',  ( 3.556430356250014579, 108.1539533981018053, 4.315625000614517148 ) ) ;
#5668=DIRECTION ( 'NONE',  ( -1.000000000000000000, -0.000000000000000000, 1.445602896647339348E-17 ) ) ;
#5669=DIRECTION ( 'NONE',  ( 1.000000000000000000, 0.000000000000000000, 0.000000000000000000 ) ) ;
#5671=CARTESIAN_POINT ( 'NONE',  ( 66.19999999999998863, 90.00000000000000000, 3.875000000000000000 ) ) ;
#5672=ORIENTED_EDGE ( 'NONE', *, *, #6843, .T. ) ;
#5673=CARTESIAN_POINT ( 'NONE',  ( 3.800000000000001155, 90.00000000000000000, -8.000000000000000000 ) ) ;
#5675=CARTESIAN_POINT ( 'NONE',  ( 5.904717470405908664, 81.90651283295660789, 1.000000000000000000 ) ) ;
#5678=EDGE_CURVE ( 'NONE', #7376, #2989, #10853, .T. ) ;
#5686=DIRECTION ( 'NONE',  ( 0.000000000000000000, 0.000000000000000000, 1.000000000000000000 ) ) ;
#5692=VERTEX_POINT ( 'NONE', #9869 ) ;
#5693=CARTESIAN_POINT ( 'NONE',  ( 66.19999999999998863, 90.00000000000000000, 4.325000000000000178 ) ) ;
#5704=AXIS2_PLACEMENT_3D ( 'NONE', #8997, #4824, #4886 ) ;
#5708=CARTESIAN_POINT ( 'NONE',  ( 35.00000000000000711, 53.69209320379640360, 3.115625000614517415 ) ) ;
#5710=CYLINDRICAL_SURFACE ( 'NONE', #2921, 31.19999999999998863 ) ;
#5715=CIRCLE ( 'NONE', #1747, 31.19999999999999218 ) ;
#5718=CARTESIAN_POINT ( 'NONE',  ( 50.72178482187499071, 117.2309300971526937, 3.809375000614517504 ) ) ;
#5726=DIRECTION ( 'NONE',  ( 0.000000000000000000, -1.000000000000000000, 0.000000000000000000 ) ) ;
#5739=DIRECTION ( 'NONE',  ( 0.000000000000000000, 0.000000000000000000, -1.000000000000000000 ) ) ;
#5740=AXIS2_PLACEMENT_3D ( 'NONE', #11891, #3132, #6853 ) ;
#5745=CARTESIAN_POINT ( 'NONE',  ( 35.00000000000000000, 90.00000000000000000, 5.000000000000000000 ) ) ;
#5765=ORIENTED_EDGE ( 'NONE', *, *, #2826, .T. ) ;
#5769=CARTESIAN_POINT ( 'NONE',  ( 19.40000000000000924, 117.0199925980744666, 4.025000000000000355 ) ) ;
#5772=CARTESIAN_POINT ( 'NONE',  ( 50.59999999999999432, 117.0199925980744666, 4.062500001229034652 ) ) ;
#5779=LINE ( 'NONE', #6952, #5968 ) ;
#5780=AXIS2_PLACEMENT_3D ( 'NONE', #7541, #5317, #11461 ) ;
#5782=CARTESIAN_POINT ( 'NONE',  ( 3.556430356250015024, 90.00000000000000000, 3.509375000614517681 ) ) ;
#5786=ORIENTED_EDGE ( 'NONE', *, *, #9657, .T. ) ;
#5788=SHAPE_REPRESENTATION_RELATIONSHIP ( 'NONE' , 'NONE' ,  #11692, #2639 ) ;
#5789=VECTOR ( 'NONE', #6682, 1000.000000000000000 ) ;
#5793=CARTESIAN_POINT ( 'NONE',  ( 19.27821517812500574, 117.2309300971526937, 3.378125000614517148 ) ) ;
#5798=CIRCLE ( 'NONE', #8924, 1.500000000000001332 ) ;
#5804=DIRECTION ( 'NONE',  ( -0.000000000000000000, 1.000000000000000000, -0.000000000000000000 ) ) ;
#5824=ORIENTED_EDGE ( 'NONE', *, *, #9479, .T. ) ;
#5827=VERTEX_POINT ( 'NONE', #5028 ) ;
#5834=CARTESIAN_POINT ( 'NONE',  ( 3.800000000000015365, 108.0133283987163111, 4.625000001229034652 ) ) ;
#5837=EDGE_CURVE ( 'NONE', #4915, #8617, #5604, .T. ) ;
#5847=CARTESIAN_POINT ( 'NONE',  ( 50.72178482187499071, 117.2309300971526937, 4.259375000614517681 ) ) ;
#5856=EDGE_CURVE ( 'NONE', #11781, #7731, #5494, .T. ) ;
#5857=CARTESIAN_POINT ( 'NONE',  ( 64.54728994471078352, 100.7543353520590870, 2.802601390178781404 ) ) ;
#5859=DIRECTION ( 'NONE',  ( -0.000000000000000000, -0.000000000000000000, -1.000000000000000000 ) ) ;
#5862=VECTOR ( 'NONE', #996, 1000.000000000000000 ) ;
#5864=DIRECTION ( 'NONE',  ( -0.000000000000000000, -0.000000000000000000, -1.000000000000000000 ) ) ;
#5876=EDGE_LOOP ( 'NONE', ( #742, #7857, #6131, #1186 ) ) ;
#5884=FACE_OUTER_BOUND ( 'NONE', #9945, .T. ) ;
#5889=CARTESIAN_POINT ( 'NONE',  ( 48.49999999999995737, 90.00000000000000000, -8.000000000000000000 ) ) ;
#5890=CARTESIAN_POINT ( 'NONE',  ( 3.800000000000015365, 90.00000000000000000, 3.312500001229034652 ) ) ;
#5892=CARTESIAN_POINT ( 'NONE',  ( 50.59999999999999432, 117.0199925980744666, 4.512500001229033941 ) ) ;
#5893=CARTESIAN_POINT ( 'NONE',  ( 5.904717470405909552, 81.90651283295660789, -1.000000000000000000 ) ) ;
#5899=ORIENTED_EDGE ( 'NONE', *, *, #11930, .F. ) ;
#5906=ADVANCED_FACE ( 'NONE', ( #12950 ), #6989, .F. ) ;
#5916=VERTEX_POINT ( 'NONE', #10324 ) ;
#5927=CIRCLE ( 'NONE', #10108, 1.500000000000001332 ) ;
#5930=AXIS2_PLACEMENT_3D ( 'NONE', #5597, #550, #11484 ) ;
#5934=ORIENTED_EDGE ( 'NONE', *, *, #11340, .T. ) ;
#5935=CARTESIAN_POINT ( 'NONE',  ( 19.40000000000002700, 62.98000740192551206, 2.937500001229034208 ) ) ;
#5941=VERTEX_POINT ( 'NONE', #5410 ) ;
#5955=CARTESIAN_POINT ( 'NONE',  ( 50.72178482187501203, 62.76906990284730625, 4.053125000614517859 ) ) ;
#5968=VECTOR ( 'NONE', #11730, 1000.000000000000000 ) ;
#5969=CARTESIAN_POINT ( 'NONE',  ( 50.72178482187501203, 62.76906990284730625, 4.109375000614517326 ) ) ;
#5974=CARTESIAN_POINT ( 'NONE',  ( 19.40000000000000924, 117.0199925980744666, 3.687500001229034208 ) ) ;
#5977=DIRECTION ( 'NONE',  ( 0.000000000000000000, -0.000000000000000000, -1.000000000000000000 ) ) ;
#5982=FACE_OUTER_BOUND ( 'NONE', #8587, .T. ) ;
#5984=FACE_OUTER_BOUND ( 'NONE', #11487, .T. ) ;
#5993=VERTEX_POINT ( 'NONE', #3400 ) ;
#5996=VECTOR ( 'NONE', #8011, 1000.000000000000000 ) ;
#6003=CARTESIAN_POINT ( 'NONE',  ( 19.40000000000002700, 62.98000740192551206, 4.174999999999999822 ) ) ;
#6006=AXIS2_PLACEMENT_3D ( 'NONE', #7532, #11385, #10538 ) ;
#6008=DIRECTION ( 'NONE',  ( 0.000000000000000000, 0.000000000000000000, -1.000000000000000000 ) ) ;
#6024=CARTESIAN_POINT ( 'NONE',  ( 3.800000000000015365, 90.00000000000000000, 3.200000000000000178 ) ) ;
#6031=EDGE_CURVE ( 'NONE', #8114, #4915, #1422, .T. ) ;
#6035=CARTESIAN_POINT ( 'NONE',  ( 50.72178482187499071, 117.2309300971526937, 3.303125000614517415 ) ) ;
#6037=VECTOR ( 'NONE', #7389, 1000.000000000000000 ) ;
#6042=CYLINDRICAL_SURFACE ( 'NONE', #1758, 1.599999999999992095 ) ;
#6060=CARTESIAN_POINT ( 'NONE',  ( 45.00000000000000000, 2.000000000000001332, 5.750000000000000888 ) ) ;
#6067=EDGE_CURVE ( 'NONE', #6209, #11848, #497, .T. ) ;
#6073=( BOUNDED_CURVE ( )  B_SPLINE_CURVE ( 2, ( #9840, #7812, #5974, #12788, #3769, #9969, #6765 ),
 .UNSPECIFIED., .F., .F. ) 
 B_SPLINE_CURVE_WITH_KNOTS ( ( 3, 2, 2, 3 ),
 ( 0.3999999999999999667, 0.4333333333333333481, 0.4666666666666667296, 0.5000000000000001110 ),
 .UNSPECIFIED. ) 
 CURVE ( )  GEOMETRIC_REPRESENTATION_ITEM ( )  RATIONAL_B_SPLINE_CURVE ( ( 1.000000000000000444, 0.8660254037844385966, 1.000000000000000000, 0.8660254037844387076, 1.000000000000000000, 0.8660254037844382635, 1.000000000000000444 ) ) 
 REPRESENTATION_ITEM ( '' )  );
#6074=EDGE_LOOP ( 'NONE', ( #7842, #495, #10728, #11018 ) ) ;
#6090=CARTESIAN_POINT ( 'NONE',  ( 66.44356964374999563, 71.84604660189820891, 4.596875000614517148 ) ) ;
#6098=CARTESIAN_POINT ( 'NONE',  ( 3.556430356250015024, 90.00000000000000000, 4.803125000614516971 ) ) ;
#6099=ORIENTED_EDGE ( 'NONE', *, *, #3712, .F. ) ;
#6115=CIRCLE ( 'NONE', #3835, 31.20000000000000284 ) ;
#6122=EDGE_LOOP ( 'NONE', ( #9284, #1495, #12007, #6640 ) ) ;
#6125=DIRECTION ( 'NONE',  ( -1.000000000000000000, 0.000000000000000000, -2.891205793294679312E-17 ) ) ;
#6131=ORIENTED_EDGE ( 'NONE', *, *, #1902, .F. ) ;
#6138=ADVANCED_FACE ( 'NONE', ( #7765 ), #8689, .T. ) ;
#6140=FACE_BOUND ( 'NONE', #2478, .T. ) ;
#6148=( BOUNDED_SURFACE ( )  B_SPLINE_SURFACE ( 1, 2, ( 
 ( #4539, #9635, #662, #1457, #9438, #3628, #11332, #4470, #2514, #6491, #10486, #1521, #5510, #8532, #8841, #3947, #7796, #6942, #982, #3754, #5955, #1721, #916, #4920, #7930, #8656, #1910, #10740, #8781, #8906, #12711, #8718, #12774, #2710, #7736, #9825, #10926, #6685, #4793, #852, #2961, #12652, #3693, #6811, #12836, #5708, #3884, #10866, #11853, #7673, #9763, #7863, #2901, #11660, #12902 ),
 ( #9695, #5834, #11790, #789, #5892, #2774, #730, #9884, #4732, #6746, #6878, #11724, #1784, #4857, #11916, #10681, #5772, #1978, #9953, #3816, #2836, #10807, #1849, #2109, #9031, #8967, #4266, #11977, #3224, #5104, #8255, #12245, #3159, #122, #4980, #3292, #12111, #2309, #10016, #3023, #11254, #4138, #1249, #8189, #8126, #11192, #5935, #10143, #4010, #4073, #7010, #6221, #10274, #7993, #7137 ) ),
 .UNSPECIFIED., .F., .F., .F. ) 
 B_SPLINE_SURFACE_WITH_KNOTS ( ( 2, 2 ),
 ( 3, 2, 2, 2, 2, 2, 2, 2, 2, 2, 2, 2, 2, 2, 2, 2, 2, 2, 2, 2, 2, 2, 2, 2, 2, 2, 2, 3 ),
 ( 0.000000000000000000, 1.000000000000000000 ),
 ( 0.000000000000000000, 0.03333333333333333287, 0.06666666666666666574, 0.1000000000000000056, 0.1333333333333333315, 0.1666666666666666574, 0.2000000000000000111, 0.2333333333333333370, 0.2666666666666666630, 0.2999999999999999889, 0.3333333333333333148, 0.3666666666666666408, 0.4000000000000000222, 0.4333333333333333481, 0.4666666666666666741, 0.5000000000000000000, 0.5333333333333333259, 0.5666666666666666519, 0.5999999999999999778, 0.6333333333333333037, 0.6666666666666666297, 0.6999999999999999556, 0.7333333333333332815, 0.7666666666666667185, 0.8000000000000000444, 0.8333333333333333703, 0.8666666666666666963, 0.8887752010635167066 ),
 .UNSPECIFIED. ) 
 GEOMETRIC_REPRESENTATION_ITEM ( )  RATIONAL_B_SPLINE_SURFACE ( (
 ( 1.000000000000000000, 0.8660254037844387076, 1.000000000000000000, 0.8660254037844387076, 1.000000000000000000, 0.8660254037844387076, 1.000000000000000000, 0.8660254037844387076, 1.000000000000000000, 0.8660254037844387076, 1.000000000000000000, 0.8660254037844387076, 1.000000000000000000, 0.8660254037844387076, 1.000000000000000000, 0.8660254037844387076, 1.000000000000000000, 0.8660254037844387076, 1.000000000000000000, 0.8660254037844387076, 1.000000000000000000, 0.8660254037844387076, 1.000000000000000000, 0.8660254037844387076, 1.000000000000000000, 0.8660254037844387076, 1.000000000000000000, 0.8660254037844387076, 1.000000000000000000, 0.8660254037844387076, 1.000000000000000000, 0.8660254037844387076, 1.000000000000000000, 0.8660254037844387076, 1.000000000000000000, 0.8660254037844387076, 1.000000000000000000, 0.8660254037844387076, 1.000000000000000000, 0.8660254037844387076, 1.000000000000000000, 0.8660254037844387076, 1.000000000000000000, 0.8660254037844387076, 1.000000000000000000, 0.8660254037844387076, 1.000000000000000000, 0.8660254037844387076, 1.000000000000000000, 0.8660254037844387076, 1.000000000000000000, 0.8660254037844387076, 1.000000000000000000, 0.9111405409379251807, 0.9401542263054123438),
 ( 1.000000000000000000, 0.8660254037844387076, 1.000000000000000000, 0.8660254037844387076, 1.000000000000000000, 0.8660254037844387076, 1.000000000000000000, 0.8660254037844387076, 1.000000000000000000, 0.8660254037844387076, 1.000000000000000000, 0.8660254037844387076, 1.000000000000000000, 0.8660254037844387076, 1.000000000000000000, 0.8660254037844387076, 1.000000000000000000, 0.8660254037844387076, 1.000000000000000000, 0.8660254037844387076, 1.000000000000000000, 0.8660254037844387076, 1.000000000000000000, 0.8660254037844387076, 1.000000000000000000, 0.8660254037844387076, 1.000000000000000000, 0.8660254037844387076, 1.000000000000000000, 0.8660254037844387076, 1.000000000000000000, 0.8660254037844387076, 1.000000000000000000, 0.8660254037844387076, 1.000000000000000000, 0.8660254037844387076, 1.000000000000000000, 0.8660254037844387076, 1.000000000000000000, 0.8660254037844387076, 1.000000000000000000, 0.8660254037844387076, 1.000000000000000000, 0.8660254037844387076, 1.000000000000000000, 0.8660254037844387076, 1.000000000000000000, 0.8660254037844387076, 1.000000000000000000, 0.8660254037844387076, 1.000000000000000000, 0.8660254037844387076, 1.000000000000000000, 0.9111405409379251807, 0.9401542263054123438) ) ) 
 REPRESENTATION_ITEM ( '' )  SURFACE ( )  );
#6151=FILL_AREA_STYLE ('',( #10991 ) ) ;
#6152=FACE_OUTER_BOUND ( 'NONE', #4124, .T. ) ;
#6154=CARTESIAN_POINT ( 'NONE',  ( 66.19999999999998863, 90.00000000000000000, 4.325000000000000178 ) ) ;
#6155=ORIENTED_EDGE ( 'NONE', *, *, #6631, .T. ) ;
#6157=CARTESIAN_POINT ( 'NONE',  ( 50.00000000000000000, 0.000000000000000000, 10.00000000000000000 ) ) ;
#6164=CARTESIAN_POINT ( 'NONE',  ( 48.49999999999995737, 90.00000000000000000, -5.000000000000000000 ) ) ;
#6166=CARTESIAN_POINT ( 'NONE',  ( 35.00000000000000711, 53.69209320379640360, 3.115625000614517415 ) ) ;
#6175=LINE ( 'NONE', #3182, #5311 ) ;
#6195=VERTEX_POINT ( 'NONE', #5675 ) ;
#6209=VERTEX_POINT ( 'NONE', #7028 ) ;
#6214=CARTESIAN_POINT ( 'NONE',  ( 25.00000000000000355, 2.000000000000000000, -5.750000000000000000 ) ) ;
#6215=DIRECTION ( 'NONE',  ( 0.000000000000000000, 0.000000000000000000, -1.000000000000000000 ) ) ;
#6220=CARTESIAN_POINT ( 'NONE',  ( 66.19999999999998863, 90.00000000000000000, 3.087500001229034119 ) ) ;
#6221=CARTESIAN_POINT ( 'NONE',  ( 35.00000000000000000, 126.0266567974326222, 2.750000001229033764 ) ) ;
#6223=LINE ( 'NONE', #4140, #10849 ) ;
#6225=CARTESIAN_POINT ( 'NONE',  ( 3.800000000000015365, 108.0133283987163111, 4.512500000000000178 ) ) ;
#6232=CARTESIAN_POINT ( 'NONE',  ( 35.00000000000000711, 53.97334320256736362, 3.762500000000000178 ) ) ;
#6235=CARTESIAN_POINT ( 'NONE',  ( 50.72178482187501203, 62.76906990284730625, 4.053125000614517859 ) ) ;
#6236=CARTESIAN_POINT ( 'NONE',  ( 35.00000000000000711, 53.69209320379639649, 4.071875000614516793 ) ) ;
#6243=LINE ( 'NONE', #5196, #6353 ) ;
#6268=EDGE_CURVE ( 'NONE', #12120, #716, #7287, .T. ) ;
#6280=AXIS2_PLACEMENT_3D ( 'NONE', #3637, #6565, #2782 ) ;
#6286=EDGE_LOOP ( 'NONE', ( #11364, #5278 ) ) ;
#6287=AXIS2_PLACEMENT_3D ( 'NONE', #6743, #10735, #9503 ) ;
#6288=CARTESIAN_POINT ( 'NONE',  ( 3.556430356250028790, 71.84604660189818048, 4.446875000614517681 ) ) ;
#6289=ORIENTED_EDGE ( 'NONE', *, *, #653, .F. ) ;
#6294=DIRECTION ( 'NONE',  ( -1.000000000000000000, 0.000000000000000000, 0.000000000000000000 ) ) ;
#6304=VECTOR ( 'NONE', #6125, 1000.000000000000000 ) ;
#6313=AXIS2_PLACEMENT_3D ( 'NONE', #11270, #12191, #3241 ) ;
#6325=VERTEX_POINT ( 'NONE', #2126 ) ;
#6330=ORIENTED_EDGE ( 'NONE', *, *, #390, .T. ) ;
#6338=VERTEX_POINT ( 'NONE', #12132 ) ;
#6340=( BOUNDED_CURVE ( )  B_SPLINE_CURVE ( 2, ( #6876, #8125, #7862, #8965, #11852, #1909, #5890 ),
 .UNSPECIFIED., .F., .F. ) 
 B_SPLINE_CURVE_WITH_KNOTS ( ( 3, 2, 2, 3 ),
 ( 0.5000000000000001110, 0.5333333333333334370, 0.5666666666666666519, 0.5999999999999999778 ),
 .UNSPECIFIED. ) 
 CURVE ( )  GEOMETRIC_REPRESENTATION_ITEM ( )  RATIONAL_B_SPLINE_CURVE ( ( 0.9999999999999995559, 0.8660254037844391517, 1.000000000000000000, 0.8660254037844387076, 1.000000000000000000, 0.8660254037844387076, 1.000000000000000000 ) ) 
 REPRESENTATION_ITEM ( '' )  );
#6349=CARTESIAN_POINT ( 'NONE',  ( 35.00000000000000711, 53.69209320379640360, 4.071875000614516793 ) ) ;
#6351=CARTESIAN_POINT ( 'NONE',  ( 20.00000000000000355, 0.000000000000000000, 1.500000000000000444 ) ) ;
#6353=VECTOR ( 'NONE', #8082, 1000.000000000000000 ) ;
#6361=EDGE_CURVE ( 'NONE', #6389, #8114, #12933, .T. ) ;
#6362=CARTESIAN_POINT ( 'NONE',  ( 66.44356964374999563, 90.00000000000000000, 3.734375000614516882 ) ) ;
#6385=DIRECTION ( 'NONE',  ( 0.000000000000000000, 0.000000000000000000, -1.000000000000000000 ) ) ;
#6386=CARTESIAN_POINT ( 'NONE',  ( 35.00000000000000000, 126.3079067962036106, 4.690625000614517148 ) ) ;
#6389=VERTEX_POINT ( 'NONE', #8534 ) ;
#6392=CARTESIAN_POINT ( 'NONE',  ( 3.800000000000015365, 90.00000000000000000, 4.662500001229034297 ) ) ;
#6394=ORIENTED_EDGE ( 'NONE', *, *, #12712, .T. ) ;
#6413=CARTESIAN_POINT ( 'NONE',  ( 3.800000000000015365, 90.00000000000000000, 4.212500001229034119 ) ) ;
#6415=ADVANCED_FACE ( 'NONE', ( #4606 ), #9507, .F. ) ;
#6422=CARTESIAN_POINT ( 'NONE',  ( 50.72178482187499071, 117.2309300971526937, 4.259375000614517681 ) ) ;
#6424=LINE ( 'NONE', #5379, #12725 ) ;
#6428=VECTOR ( 'NONE', #10359, 1000.000000000000000 ) ;
#6430=EDGE_CURVE ( 'NONE', #8420, #427, #6424, .T. ) ;
#6449=FACE_OUTER_BOUND ( 'NONE', #3648, .T. ) ;
#6450=ORIENTED_EDGE ( 'NONE', *, *, #5037, .T. ) ;
#6456=CIRCLE ( 'NONE', #1665, 4.999999999999997335 ) ;
#6470=( NAMED_UNIT ( * ) PLANE_ANGLE_UNIT ( ) SI_UNIT ( $, .RADIAN. ) );
#6474=DIRECTION ( 'NONE',  ( -0.8660254037844365982, -0.5000000000000036637, 0.000000000000000000 ) ) ;
#6478=FACE_OUTER_BOUND ( 'NONE', #1972, .T. ) ;
#6481=CARTESIAN_POINT ( 'NONE',  ( 66.44356964374999563, 90.00000000000000000, 4.184375000614516615 ) ) ;
#6488=CARTESIAN_POINT ( 'NONE',  ( 3.799999999999985612, 108.0133283987162827, 4.062500000000000000 ) ) ;
#6490=CARTESIAN_POINT ( 'NONE',  ( 19.27821517812500574, 117.2309300971526937, 2.984375000614517326 ) ) ;
#6491=CARTESIAN_POINT ( 'NONE',  ( 35.00000000000000711, 53.69209320379640360, 4.465625000614517504 ) ) ;
#6508=DIRECTION ( 'NONE',  ( -0.000000000000000000, -0.000000000000000000, -1.000000000000000000 ) ) ;
#6524=CARTESIAN_POINT ( 'NONE',  ( 40.00000000000000000, 0.000000000000000000, 10.00000000000000000 ) ) ;
#6525=ORIENTED_EDGE ( 'NONE', *, *, #2882, .T. ) ;
#6535=ORIENTED_EDGE ( 'NONE', *, *, #7511, .T. ) ;
#6538=VERTEX_POINT ( 'NONE', #12238 ) ;
#6544=CARTESIAN_POINT ( 'NONE',  ( 66.44356964374999563, 71.84604660189820891, 3.246875000614517059 ) ) ;
#6546=LINE ( 'NONE', #5570, #3966 ) ;
#6565=DIRECTION ( 'NONE',  ( 0.000000000000000000, 0.000000000000000000, 1.000000000000000000 ) ) ;
#6567=ORIENTED_EDGE ( 'NONE', *, *, #8645, .F. ) ;
#6570=CIRCLE ( 'NONE', #5740, 4.999999999999997335 ) ;
#6571=AXIS2_PLACEMENT_3D ( 'NONE', #2441, #2373, #9363 ) ;
#6578=DIRECTION ( 'NONE',  ( -0.000000000000000000, -0.000000000000000000, -1.000000000000000000 ) ) ;
#6580=ORIENTED_EDGE ( 'NONE', *, *, #12762, .F. ) ;
#6583=EDGE_LOOP ( 'NONE', ( #11821, #7904 ) ) ;
#6589=CARTESIAN_POINT ( 'NONE',  ( 50.59999999999999432, 117.0199925980744666, 4.400000000000000355 ) ) ;
#6591=ORIENTED_EDGE ( 'NONE', *, *, #3401, .F. ) ;
#6598=EDGE_LOOP ( 'NONE', ( #3608, #45, #7380, #9141 ) ) ;
#6610=CARTESIAN_POINT ( 'NONE',  ( 35.00000000000000711, 53.97334320256736362, 4.325000001229033941 ) ) ;
#6612=FACE_OUTER_BOUND ( 'NONE', #12750, .T. ) ;
#6617=CARTESIAN_POINT ( 'NONE',  ( 30.00000000000000711, 2.000000000000000000, 10.00000000000000000 ) ) ;
#6622=ADVANCED_FACE ( 'NONE', ( #7197 ), #10338, .F. ) ;
#6631=EDGE_CURVE ( 'NONE', #9145, #2190, #11249, .T. ) ;
#6635=VERTEX_POINT ( 'NONE', #10268 ) ;
#6639=LINE ( 'NONE', #2665, #4467 ) ;
#6640=ORIENTED_EDGE ( 'NONE', *, *, #2870, .T. ) ;
#6643=CARTESIAN_POINT ( 'NONE',  ( 66.44356964374998142, 108.1539533981018053, 3.265625000614517326 ) ) ;
#6681=LINE ( 'NONE', #786, #10473 ) ;
#6682=DIRECTION ( 'NONE',  ( -0.000000000000000000, -0.000000000000000000, 1.000000000000000000 ) ) ;
#6683=EDGE_CURVE ( 'NONE', #767, #9108, #2712, .T. ) ;
#6685=CARTESIAN_POINT ( 'NONE',  ( 3.556430356250014579, 108.1539533981018053, 3.415625000614517237 ) ) ;
#6693=CARTESIAN_POINT ( 'NONE',  ( 50.00000000000000000, 2.000000000000001776, -1.500000000000000000 ) ) ;
#6694=CARTESIAN_POINT ( 'NONE',  ( 19.27821517812500574, 117.2309300971526937, 4.784375000614516260 ) ) ;
#6703=EDGE_CURVE ( 'NONE', #1821, #5315, #1594, .T. ) ;
#6707=CARTESIAN_POINT ( 'NONE',  ( 40.00000000000000000, 2.000000000000000000, -10.00000000000000000 ) ) ;
#6717=CARTESIAN_POINT ( 'NONE',  ( 66.19999999999998863, 90.00000000000000000, 3.987500001229034030 ) ) ;
#6718=LINE ( 'NONE', #2806, #4675 ) ;
#6723=DIRECTION ( 'NONE',  ( -0.000000000000000000, 1.000000000000000000, -0.000000000000000000 ) ) ;
#6725=CARTESIAN_POINT ( 'NONE',  ( 35.00000000000000000, 90.00000000000000000, 1.000000000000000000 ) ) ;
#6728=VERTEX_POINT ( 'NONE', #8535 ) ;
#6732=CARTESIAN_POINT ( 'NONE',  ( 3.800000000000015365, 90.00000000000000000, 5.000000000000000000 ) ) ;
#6738=CARTESIAN_POINT ( 'NONE',  ( 25.00000000000000355, 2.000000000000001332, -4.150000000000012790 ) ) ;
#6741=EDGE_CURVE ( 'NONE', #7595, #1608, #1659, .T. ) ;
#6743=CARTESIAN_POINT ( 'NONE',  ( 30.00000000000000711, 0.000000000000000000, 10.00000000000000000 ) ) ;
#6746=CARTESIAN_POINT ( 'NONE',  ( 35.00000000000000711, 53.97334320256736362, 4.325000001229033941 ) ) ;
#6761=CARTESIAN_POINT ( 'NONE',  ( 50.72178482187499071, 117.2309300971526937, 2.909375000614517148 ) ) ;
#6765=CARTESIAN_POINT ( 'NONE',  ( 66.19999999999998863, 90.00000000000000000, 3.537500001229034297 ) ) ;
#6771=EDGE_CURVE ( 'NONE', #4991, #12815, #6456, .T. ) ;
#6773=CARTESIAN_POINT ( 'NONE',  ( 12.66025403784434822, 85.80682368868758658, 1.000000000000000000 ) ) ;
#6774=CARTESIAN_POINT ( 'NONE',  ( 3.556430356250015024, 90.00000000000000000, 3.903125000614517504 ) ) ;
#6779=FACE_BOUND ( 'NONE', #8683, .T. ) ;
#6783=LINE ( 'NONE', #10779, #8015 ) ;
#6800=ORIENTED_EDGE ( 'NONE', *, *, #1425, .F. ) ;
#6810=CARTESIAN_POINT ( 'NONE',  ( 25.00000000000000355, 0.000000000000000000, -5.750000000000000000 ) ) ;
#6811=CARTESIAN_POINT ( 'NONE',  ( 66.44356964374999563, 71.84604660189820891, 3.190625000614517592 ) ) ;
#6817=DIRECTION ( 'NONE',  ( -0.000000000000000000, -0.000000000000000000, -1.000000000000000000 ) ) ;
#6823=CARTESIAN_POINT ( 'NONE',  ( 66.44356964374998142, 108.1539533981018053, 3.321875000614517237 ) ) ;
#6824=ORIENTED_EDGE ( 'NONE', *, *, #2826, .F. ) ;
#6835=CARTESIAN_POINT ( 'NONE',  ( 35.00000000000000000, 126.3079067962036106, 2.890625000614516882 ) ) ;
#6843=EDGE_CURVE ( 'NONE', #12533, #1608, #8719, .T. ) ;
#6853=DIRECTION ( 'NONE',  ( -1.000000000000000000, 0.000000000000000000, 0.000000000000000000 ) ) ;
#6876=CARTESIAN_POINT ( 'NONE',  ( 66.19999999999998863, 90.00000000000000000, 3.537500001229034297 ) ) ;
#6878=CARTESIAN_POINT ( 'NONE',  ( 19.40000000000002700, 62.98000740192551206, 4.287500001229034297 ) ) ;
#6891=CARTESIAN_POINT ( 'NONE',  ( 19.27821517812503060, 62.76906990284727783, 3.584375000614516971 ) ) ;
#6899=ADVANCED_FACE ( 'NONE', ( #918 ), #2713, .T. ) ;
#6900=CARTESIAN_POINT ( 'NONE',  ( 64.54728993811707483, 100.7543353701752125, 2.858851390224067313 ) ) ;
#6903=LINE ( 'NONE', #14, #12885 ) ;
#6906=PLANE ( 'NONE',  #2458 ) ;
#6914=CARTESIAN_POINT ( 'NONE',  ( 30.00000000000000711, 121.2009999999999934, -1.499999999999999778 ) ) ;
#6922=VERTEX_POINT ( 'NONE', #5893 ) ;
#6925=ORIENTED_EDGE ( 'NONE', *, *, #2532, .T. ) ;
#6931=FACE_BOUND ( 'NONE', #652, .T. ) ;
#6933=DIRECTION ( 'NONE',  ( 0.000000000000000000, -0.000000000000000000, -1.000000000000000000 ) ) ;
#6935=ORIENTED_EDGE ( 'NONE', *, *, #12308, .F. ) ;
#6938=FACE_OUTER_BOUND ( 'NONE', #8192, .T. ) ;
#6942=CARTESIAN_POINT ( 'NONE',  ( 66.44356964374998142, 108.1539533981018053, 4.165625000614516793 ) ) ;
#6943=ADVANCED_FACE ( 'NONE', ( #7798 ), #5710, .T. ) ;
#6945=B_SPLINE_CURVE_WITH_KNOTS ( 'NONE', 3,
 ( #6900, #1006, #12860, #8802 ),
 .UNSPECIFIED., .F., .F.,
 ( 4, 4 ),
 ( 0.000000000000000000, 1.000000000000000000 ),
 .UNSPECIFIED. ) ;
#6950=ORIENTED_EDGE ( 'NONE', *, *, #9902, .T. ) ;
#6952=CARTESIAN_POINT ( 'NONE',  ( 50.00000000000000000, 0.000000000000000000, 10.00000000000000000 ) ) ;
#6955=CARTESIAN_POINT ( 'NONE',  ( 3.556430356250015024, 90.00000000000000000, 3.959375000614517415 ) ) ;
#6960=EDGE_CURVE ( 'NONE', #6922, #9462, #6223, .T. ) ;
#6963=VECTOR ( 'NONE', #8181, 1000.000000000000000 ) ;
#6964=DIRECTION ( 'NONE',  ( -0.000000000000000000, 1.000000000000000000, -0.000000000000000000 ) ) ;
#6966=CARTESIAN_POINT ( 'NONE',  ( 66.19999999999998863, 90.00000000000000000, 5.000000000000000000 ) ) ;
#6969=CARTESIAN_POINT ( 'NONE',  ( 64.31840976852106451, 100.6710284717588024, 2.999476386674974737 ) ) ;
#6971=DIRECTION ( 'NONE',  ( 1.000000000000000000, -0.000000000000000000, -0.000000000000000000 ) ) ;
#6989=CYLINDRICAL_SURFACE ( 'NONE', #4574, 1.599999999999992095 ) ;
#6997=VERTEX_POINT ( 'NONE', #11980 ) ;
#7003=DIRECTION ( 'NONE',  ( 0.000000000000000000, -1.000000000000000000, 0.000000000000000000 ) ) ;
#7010=CARTESIAN_POINT ( 'NONE',  ( 19.40000000000000924, 117.0199925980744666, 2.787500001229034297 ) ) ;
#7015=CARTESIAN_POINT ( 'NONE',  ( 64.31840934454761793, 100.6710296366163249, 2.999476389609550431 ) ) ;
#7022=CARTESIAN_POINT ( 'NONE',  ( 35.00000000000000711, 53.69209320379640360, 4.465625000614517504 ) ) ;
#7028=CARTESIAN_POINT ( 'NONE',  ( 40.00000000000000000, 2.000000000000000000, 10.00000000000000000 ) ) ;
#7041=LINE ( 'NONE', #8935, #9880 ) ;
#7049=ORIENTED_EDGE ( 'NONE', *, *, #9072, .F. ) ;
#7055=CARTESIAN_POINT ( 'NONE',  ( 19.99999999999998224, 90.00000000000000000, -8.000000000000000000 ) ) ;
#7064=ORIENTED_EDGE ( 'NONE', *, *, #9484, .F. ) ;
#7065=DIRECTION ( 'NONE',  ( -0.000000000000000000, 1.000000000000000000, -0.000000000000000000 ) ) ;
#7069=CYLINDRICAL_SURFACE ( 'NONE', #5, 1.500000000000001332 ) ;
#7071=ADVANCED_FACE ( 'NONE', ( #6152 ), #8128, .F. ) ;
#7077=ORIENTED_EDGE ( 'NONE', *, *, #2035, .T. ) ;
#7078=CARTESIAN_POINT ( 'NONE',  ( 50.60000000000001563, 62.98000740192552627, 3.350000000000000533 ) ) ;
#7082=CARTESIAN_POINT ( 'NONE',  ( 66.19999999999998863, 90.00000000000000000, 3.875000000000000000 ) ) ;
#7088=CARTESIAN_POINT ( 'NONE',  ( 66.44356964374999563, 71.84604660189820891, 4.090625000614517504 ) ) ;
#7095=CYLINDRICAL_SURFACE ( 'NONE', #3653, 1.599999999999993872 ) ;
#7096=DIRECTION ( 'NONE',  ( -0.000000000000000000, 1.000000000000000000, -0.000000000000000000 ) ) ;
#7098=CARTESIAN_POINT ( 'NONE',  ( 19.99999999999998224, 90.00000000000000000, -5.000000000000000000 ) ) ;
#7099=DIRECTION ( 'NONE',  ( -1.000000000000000000, 0.000000000000000000, -2.891205793294679312E-17 ) ) ;
#7107=CARTESIAN_POINT ( 'NONE',  ( 45.00000000000000000, 0.000000000000000000, -5.750000000000000000 ) ) ;
#7111=ORIENTED_EDGE ( 'NONE', *, *, #5011, .T. ) ;
#7126=CARTESIAN_POINT ( 'NONE',  ( 10.16381611175368604, 72.81849919625140899, 1.000000000000000000 ) ) ;
#7130=VERTEX_POINT ( 'NONE', #6717 ) ;
#7137=CARTESIAN_POINT ( 'NONE',  ( 64.31840935109022439, 100.6710296186405600, 2.661976390793298286 ) ) ;
#7141=CARTESIAN_POINT ( 'NONE',  ( 3.800000000000015365, 90.00000000000000000, 3.650000000000000355 ) ) ;
#7142=EDGE_CURVE ( 'NONE', #2989, #7686, #7497, .T. ) ;
#7143=DIRECTION ( 'NONE',  ( -0.000000000000000000, 1.000000000000000000, -0.000000000000000000 ) ) ;
#7146=CYLINDRICAL_SURFACE ( 'NONE', #54, 1.599999999999993872 ) ;
#7150=CARTESIAN_POINT ( 'NONE',  ( 3.556430356250015024, 90.00000000000000000, 4.803125000614516971 ) ) ;
#7156=CIRCLE ( 'NONE', #1937, 1.599999999999997202 ) ;
#7160=DIRECTION ( 'NONE',  ( -1.000000000000000000, 0.000000000000000000, 0.000000000000000000 ) ) ;
#7161=CARTESIAN_POINT ( 'NONE',  ( 20.00000000000000355, 62.64236852357281293, 1.500000000000000444 ) ) ;
#7168=VECTOR ( 'NONE', #2744, 1000.000000000000000 ) ;
#7190=AXIS2_PLACEMENT_3D ( 'NONE', #9392, #414, #2210 ) ;
#7192=ORIENTED_EDGE ( 'NONE', *, *, #8910, .T. ) ;
#7197=FACE_OUTER_BOUND ( 'NONE', #4360, .T. ) ;
#7205=CARTESIAN_POINT ( 'NONE',  ( 19.40000000000002700, 62.98000740192551206, 4.625000000000000000 ) ) ;
#7209=ORIENTED_EDGE ( 'NONE', *, *, #12475, .T. ) ;
#7210=CARTESIAN_POINT ( 'NONE',  ( 35.00000000000000711, 53.97334320256736362, 4.662499999999999645 ) ) ;
#7219=CARTESIAN_POINT ( 'NONE',  ( 66.44356964374999563, 71.84604660189820891, 4.540625000614517681 ) ) ;
#7220=CARTESIAN_POINT ( 'NONE',  ( 66.44356964374999563, 90.00000000000000000, 4.184375000614516615 ) ) ;
#7229=LINE ( 'NONE', #1269, #4475 ) ;
#7241=CARTESIAN_POINT ( 'NONE',  ( 20.00000000000000355, 2.000000000000001776, 1.500000000000000444 ) ) ;
#7242=DIRECTION ( 'NONE',  ( 0.000000000000000000, 0.000000000000000000, 1.000000000000000000 ) ) ;
#7245=CARTESIAN_POINT ( 'NONE',  ( 10.16381611175368604, 72.81849919625140899, 5.000000000000000000 ) ) ;
#7246=CARTESIAN_POINT ( 'NONE',  ( 66.19999999999998863, 90.00000000000000000, 3.987500001229034030 ) ) ;
#7252=ORIENTED_EDGE ( 'NONE', *, *, #1929, .F. ) ;
#7256=ORIENTED_EDGE ( 'NONE', *, *, #7600, .F. ) ;
#7265=EDGE_CURVE ( 'NONE', #427, #10175, #7418, .T. ) ;
#7266=( BOUNDED_CURVE ( )  B_SPLINE_CURVE ( 2, ( #1196, #9900, #932, #2058, #10031, #1061, #8270, #1262, #12382, #9436, #8335, #8464, #10484, #5255, #2260, #8399, #6422, #1456, #7220, #460, #2324, #6236, #5443, #11208, #2383, #9243, #1520, #2450, #10358, #11331, #6362, #12260, #7412, #3307, #4469, #4282, #10421, #10290, #10228, #12452, #11399, #3499, #7478, #4343, #1390, #11462, #396, #2513, #8205, #265, #6490, #5509, #334, #7285, #12323 ),
 .UNSPECIFIED., .F., .F. ) 
 B_SPLINE_CURVE_WITH_KNOTS ( ( 3, 2, 2, 2, 2, 2, 2, 2, 2, 2, 2, 2, 2, 2, 2, 2, 2, 2, 2, 2, 2, 2, 2, 2, 2, 2, 2, 3 ),
 ( 0.000000000000000000, 0.03333333333333333287, 0.06666666666666666574, 0.1000000000000000056, 0.1333333333333333315, 0.1666666666666666574, 0.2000000000000000111, 0.2333333333333333370, 0.2666666666666666630, 0.2999999999999999889, 0.3333333333333333148, 0.3666666666666666408, 0.4000000000000000222, 0.4333333333333333481, 0.4666666666666666741, 0.5000000000000000000, 0.5333333333333333259, 0.5666666666666666519, 0.5999999999999999778, 0.6333333333333333037, 0.6666666666666666297, 0.6999999999999999556, 0.7333333333333332815, 0.7666666666666667185, 0.8000000000000000444, 0.8333333333333333703, 0.8666666666666666963, 0.8887752010443025208 ),
 .UNSPECIFIED. ) 
 CURVE ( )  GEOMETRIC_REPRESENTATION_ITEM ( )  RATIONAL_B_SPLINE_CURVE ( ( 1.000000000000000000, 0.8660254037844387076, 1.000000000000000000, 0.8660254037844387076, 1.000000000000000000, 0.8660254037844387076, 1.000000000000000000, 0.8660254037844387076, 1.000000000000000000, 0.8660254037844387076, 1.000000000000000000, 0.8660254037844387076, 1.000000000000000000, 0.8660254037844387076, 1.000000000000000000, 0.8660254037844387076, 1.000000000000000000, 0.8660254037844387076, 1.000000000000000000, 0.8660254037844387076, 1.000000000000000000, 0.8660254037844387076, 1.000000000000000000, 0.8660254037844387076, 1.000000000000000000, 0.8660254037844387076, 1.000000000000000000, 0.8660254037844387076, 1.000000000000000000, 0.8660254037844387076, 1.000000000000000000, 0.8660254037844387076, 1.000000000000000000, 0.8660254037844387076, 1.000000000000000000, 0.8660254037844387076, 1.000000000000000000, 0.8660254037844387076, 1.000000000000000000, 0.8660254037844387076, 1.000000000000000000, 0.8660254037844387076, 1.000000000000000000, 0.8660254037844387076, 1.000000000000000000, 0.8660254037844387076, 1.000000000000000000, 0.8660254037844387076, 1.000000000000000000, 0.8660254037844387076, 1.000000000000000000, 0.8660254037844387076, 1.000000000000000000, 0.9111405410151519613, 0.9401542262549813511 ) ) 
 REPRESENTATION_ITEM ( '' )  );
#7272=EDGE_CURVE ( 'NONE', #9145, #9386, #1001, .T. ) ;
#7273=ORIENTED_EDGE ( 'NONE', *, *, #4413, .T. ) ;
#7275=CARTESIAN_POINT ( 'NONE',  ( 66.20000000000000284, 71.98667160128370313, 3.387500000000000178 ) ) ;
#7285=CARTESIAN_POINT ( 'NONE',  ( 60.63303221600038739, 111.5086687461494250, 2.885734441893565538 ) ) ;
#7287=LINE ( 'NONE', #3373, #3325 ) ;
#7291=DIRECTION ( 'NONE',  ( 0.000000000000000000, 0.000000000000000000, -1.000000000000000000 ) ) ;
#7293=CARTESIAN_POINT ( 'NONE',  ( 20.00000000000000355, 0.000000000000000000, -10.00000000000000000 ) ) ;
#7311=CIRCLE ( 'NONE', #1673, 30.19999999999999218 ) ;
#7313=EDGE_LOOP ( 'NONE', ( #657, #3385, #4112, #8855 ) ) ;
#7315=CARTESIAN_POINT ( 'NONE',  ( 50.59999999999999432, 117.0199925980744666, 4.512500001229033941 ) ) ;
#7319=ADVANCED_FACE ( 'NONE', ( #4040 ), #11945, .F. ) ;
#7326=ORIENTED_EDGE ( 'NONE', *, *, #8839, .T. ) ;
#7329=AXIS2_PLACEMENT_3D ( 'NONE', #9240, #458, #4466 ) ;
#7331=CARTESIAN_POINT ( 'NONE',  ( 3.800000000000015810, 108.0133283987162969, 3.275000001229034563 ) ) ;
#7338=CARTESIAN_POINT ( 'NONE',  ( 50.72178482187499071, 117.2309300971526937, 3.809375000614517504 ) ) ;
#7351=DIRECTION ( 'NONE',  ( -0.000000000000000000, -0.000000000000000000, -1.000000000000000000 ) ) ;
#7354=DIRECTION ( 'NONE',  ( -0.5000000000000036637, 0.8660254037844365982, 0.000000000000000000 ) ) ;
#7376=VERTEX_POINT ( 'NONE', #10896 ) ;
#7377=CARTESIAN_POINT ( 'NONE',  ( 64.31840935109022439, 100.6710296186405742, 2.661976390793298286 ) ) ;
#7380=ORIENTED_EDGE ( 'NONE', *, *, #6771, .F. ) ;
#7385=AXIS2_PLACEMENT_3D ( 'NONE', #10284, #1316, #5312 ) ;
#7387=CARTESIAN_POINT ( 'NONE',  ( 50.60000000000001563, 62.98000740192552627, 3.350000000000000533 ) ) ;
#7389=DIRECTION ( 'NONE',  ( -0.000000000000000000, 1.000000000000000000, -0.000000000000000000 ) ) ;
#7402=CARTESIAN_POINT ( 'NONE',  ( 50.72178482187501203, 62.76906990284730625, 3.209375000614517415 ) ) ;
#7403=ORIENTED_EDGE ( 'NONE', *, *, #11304, .T. ) ;
#7407=ORIENTED_EDGE ( 'NONE', *, *, #2025, .F. ) ;
#7412=CARTESIAN_POINT ( 'NONE',  ( 50.72178482187501203, 62.76906990284730625, 3.659375000614517592 ) ) ;
#7418=( BOUNDED_CURVE ( )  B_SPLINE_CURVE ( 2, ( #2078, #1014, #12873, #5012, #3979, #1941, #4105 ),
 .UNSPECIFIED., .F., .F. ) 
 B_SPLINE_CURVE_WITH_KNOTS ( ( 3, 2, 2, 3 ),
 ( 0.5999999999999999778, 0.6333333333333334147, 0.6666666666666667407, 0.7000000000000001776 ),
 .UNSPECIFIED. ) 
 CURVE ( )  GEOMETRIC_REPRESENTATION_ITEM ( )  RATIONAL_B_SPLINE_CURVE ( ( 1.000000000000000000, 0.8660254037844387076, 1.000000000000000000, 0.8660254037844387076, 1.000000000000000000, 0.8660254037844378194, 1.000000000000000888 ) ) 
 REPRESENTATION_ITEM ( '' )  );
#7425=DIRECTION ( 'NONE',  ( -0.000000000000000000, -0.000000000000000000, -1.000000000000000000 ) ) ;
#7433=FACE_OUTER_BOUND ( 'NONE', #1041, .T. ) ;
#7437=EDGE_CURVE ( 'NONE', #6538, #4251, #2140, .T. ) ;
#7440=CARTESIAN_POINT ( 'NONE',  ( 3.556430356250015024, 90.00000000000000000, 4.803125000614516971 ) ) ;
#7445=DIRECTION ( 'NONE',  ( 0.000000000000000000, 0.000000000000000000, 1.000000000000000000 ) ) ;
#7463=CARTESIAN_POINT ( 'NONE',  ( 3.800000000000015365, 90.00000000000000000, 3.312500001229034652 ) ) ;
#7467=CARTESIAN_POINT ( 'NONE',  ( 35.00000000000000000, 126.3079067962035822, 4.296875000614517326 ) ) ;
#7470=CARTESIAN_POINT ( 'NONE',  ( 35.00000000000000711, 53.97334320256736362, 2.975000001229034297 ) ) ;
#7478=CARTESIAN_POINT ( 'NONE',  ( 66.44356964374999563, 90.00000000000000000, 3.284375000614517148 ) ) ;
#7497=( BOUNDED_CURVE ( )  B_SPLINE_CURVE ( 2, ( #1626, #10278, #763, #7766, #6589, #10711, #1557 ),
 .UNSPECIFIED., .F., .F. ) 
 B_SPLINE_CURVE_WITH_KNOTS ( ( 3, 2, 2, 3 ),
 ( 0.1999999999999999833, 0.2333333333333333925, 0.2666666666666668295, 0.3000000000000002109 ),
 .UNSPECIFIED. ) 
 CURVE ( )  GEOMETRIC_REPRESENTATION_ITEM ( )  RATIONAL_B_SPLINE_CURVE ( ( 1.000000000000000222, 0.8660254037844385966, 1.000000000000000000, 0.8660254037844387076, 1.000000000000000000, 0.8660254037844378194, 1.000000000000000888 ) ) 
 REPRESENTATION_ITEM ( '' )  );
#7500=EDGE_CURVE ( 'NONE', #3935, #6325, #11351, .T. ) ;
#7501=DIRECTION ( 'NONE',  ( -1.000000000000000000, 0.000000000000000000, 0.000000000000000000 ) ) ;
#7502=ORIENTED_EDGE ( 'NONE', *, *, #2802, .F. ) ;
#7505=ORIENTED_EDGE ( 'NONE', *, *, #7925, .F. ) ;
#7509=CARTESIAN_POINT ( 'NONE',  ( 3.800000000000015365, 90.00000000000000000, 2.862500001229034474 ) ) ;
#7511=EDGE_CURVE ( 'NONE', #12815, #4991, #7815, .T. ) ;
#7513=CARTESIAN_POINT ( 'NONE',  ( 65.19999999999998863, 90.00000000000000000, 5.000000000000000000 ) ) ;
#7527=ORIENTED_EDGE ( 'NONE', *, *, #12466, .T. ) ;
#7532=CARTESIAN_POINT ( 'NONE',  ( 20.00000000000000355, 121.2009999999999934, -1.499999999999999556 ) ) ;
#7541=CARTESIAN_POINT ( 'NONE',  ( 30.00000000000000711, 0.000000000000000000, 10.00000000000000000 ) ) ;
#7545=AXIS2_PLACEMENT_3D ( 'NONE', #6164, #1454, #6294 ) ;
#7573=CARTESIAN_POINT ( 'NONE',  ( 25.00000000000000355, 0.000000000000000000, -7.349999999999996980 ) ) ;
#7581=FACE_OUTER_BOUND ( 'NONE', #8745, .T. ) ;
#7582=VERTEX_POINT ( 'NONE', #11549 ) ;
#7595=VERTEX_POINT ( 'NONE', #2533 ) ;
#7596=CARTESIAN_POINT ( 'NONE',  ( 50.72178482187499071, 117.2309300971526937, 2.909375000614517148 ) ) ;
#7599=FACE_OUTER_BOUND ( 'NONE', #12667, .T. ) ;
#7600=EDGE_CURVE ( 'NONE', #307, #5827, #9526, .T. ) ;
#7630=DIRECTION ( 'NONE',  ( 0.5000000000000036637, -0.8660254037844365982, 0.000000000000000000 ) ) ;
#7631=CARTESIAN_POINT ( 'NONE',  ( 66.44356964374999563, 90.00000000000000000, 4.128125000614517148 ) ) ;
#7637=DIRECTION ( 'NONE',  ( -0.000000000000000000, -0.000000000000000000, -1.000000000000000000 ) ) ;
#7650=ADVANCED_FACE ( 'NONE', ( #8675 ), #9455, .T. ) ;
#7651=ORIENTED_EDGE ( 'NONE', *, *, #9484, .T. ) ;
#7659=UNCERTAINTY_MEASURE_WITH_UNIT (LENGTH_MEASURE( 1.000000000000000082E-05 ), #2044, 'distance_accuracy_value', 'NONE');
#7662=LINE ( 'NONE', #1709, #9720 ) ;
#7664=CARTESIAN_POINT ( 'NONE',  ( 3.800000000000015365, 90.00000000000000000, 2.862500001229034474 ) ) ;
#7673=CARTESIAN_POINT ( 'NONE',  ( 3.556430356250014579, 108.1539533981018053, 2.965625000614517504 ) ) ;
#7677=CARTESIAN_POINT ( 'NONE',  ( 3.800000000000055334, 71.98667160128364628, 3.800000001229034474 ) ) ;
#7684=LINE ( 'NONE', #12722, #847 ) ;
#7685=CARTESIAN_POINT ( 'NONE',  ( 3.556430356250028790, 71.84604660189818048, 3.546875000614516882 ) ) ;
#7686=VERTEX_POINT ( 'NONE', #10696 ) ;
#7698=CARTESIAN_POINT ( 'NONE',  ( 20.00000000000000355, 0.000000000000000000, -1.499999999999999556 ) ) ;
#7700=EDGE_LOOP ( 'NONE', ( #8441, #12251, #10579, #2530 ) ) ;
#7705=ADVANCED_FACE ( 'NONE', ( #7816 ), #6042, .F. ) ;
#7712=DIRECTION ( 'NONE',  ( -1.000000000000000000, 0.000000000000000000, 0.000000000000000000 ) ) ;
#7719=ORIENTED_EDGE ( 'NONE', *, *, #11408, .T. ) ;
#7728=CARTESIAN_POINT ( 'NONE',  ( 0.000000000000000000, 0.000000000000000000, 0.000000000000000000 ) ) ;
#7729=ORIENTED_EDGE ( 'NONE', *, *, #9817, .F. ) ;
#7731=VERTEX_POINT ( 'NONE', #12000 ) ;
#7736=CARTESIAN_POINT ( 'NONE',  ( 19.27821517812503060, 62.76906990284727783, 3.528125000614517059 ) ) ;
#7744=CYLINDRICAL_SURFACE ( 'NONE', #948, 31.19999999999998863 ) ;
#7746=CARTESIAN_POINT ( 'NONE',  ( 50.72178482187499071, 117.2309300971526937, 3.359375000614517326 ) ) ;
#7757=CARTESIAN_POINT ( 'NONE',  ( 19.27821517812503060, 62.76906990284727783, 3.078125000614517326 ) ) ;
#7765=FACE_OUTER_BOUND ( 'NONE', #2851, .T. ) ;
#7766=CARTESIAN_POINT ( 'NONE',  ( 35.00000000000000000, 126.0266567974326222, 4.437500000000000888 ) ) ;
#7776=ORIENTED_EDGE ( 'NONE', *, *, #756, .F. ) ;
#7783=CIRCLE ( 'NONE', #12176, 1.500000000000001332 ) ;
#7787=PLANE ( 'NONE',  #10015 ) ;
#7792=CARTESIAN_POINT ( 'NONE',  ( 20.00000000000000355, 2.000000000000000000, 10.00000000000000000 ) ) ;
#7796=CARTESIAN_POINT ( 'NONE',  ( 50.72178482187499071, 117.2309300971526937, 4.203125000614517326 ) ) ;
#7798=FACE_OUTER_BOUND ( 'NONE', #1879, .T. ) ;
#7808=CARTESIAN_POINT ( 'NONE',  ( 66.44356964374998142, 108.1539533981018053, 4.671875000614516438 ) ) ;
#7812=CARTESIAN_POINT ( 'NONE',  ( 3.799999999999985612, 108.0133283987162827, 3.725000001229034741 ) ) ;
#7815=CIRCLE ( 'NONE', #7190, 4.999999999999997335 ) ;
#7816=FACE_OUTER_BOUND ( 'NONE', #9815, .T. ) ;
#7819=CARTESIAN_POINT ( 'NONE',  ( 3.556430356250028790, 71.84604660189818048, 3.490625000614516971 ) ) ;
#7832=LINE ( 'NONE', #1015, #12811 ) ;
#7833=CIRCLE ( 'NONE', #4294, 4.999999999999997335 ) ;
#7842=ORIENTED_EDGE ( 'NONE', *, *, #6960, .F. ) ;
#7845=ORIENTED_EDGE ( 'NONE', *, *, #6703, .F. ) ;
#7855=DIRECTION ( 'NONE',  ( 0.000000000000000000, 0.000000000000000000, 1.000000000000000000 ) ) ;
#7857=ORIENTED_EDGE ( 'NONE', *, *, #6031, .T. ) ;
#7861=CARTESIAN_POINT ( 'NONE',  ( 3.800000000000015365, 90.00000000000000000, 3.200000000000000178 ) ) ;
#7862=CARTESIAN_POINT ( 'NONE',  ( 50.60000000000001563, 62.98000740192552627, 3.462500001229034563 ) ) ;
#7863=CARTESIAN_POINT ( 'NONE',  ( 35.00000000000000000, 126.3079067962035822, 2.890625000614516882 ) ) ;
#7868=CARTESIAN_POINT ( 'NONE',  ( 19.40000000000000924, 117.0199925980744666, 4.924999999999999822 ) ) ;
#7878=CARTESIAN_POINT ( 'NONE',  ( 35.00000000000000711, 53.69209320379640360, 4.521875000614516971 ) ) ;
#7882=ORIENTED_EDGE ( 'NONE', *, *, #7437, .T. ) ;
#7887=CARTESIAN_POINT ( 'NONE',  ( 20.00000000000000355, 2.000000000000000000, 10.00000000000000000 ) ) ;
#7890=CYLINDRICAL_SURFACE ( 'NONE', #9750, 31.19999999999998863 ) ;
#7896=ADVANCED_FACE ( 'NONE', ( #4349, #12328 ), #5060, .T. ) ;
#7904=ORIENTED_EDGE ( 'NONE', *, *, #7272, .T. ) ;
#7912=AXIS2_PLACEMENT_3D ( 'NONE', #821, #8012, #12682 ) ;
#7914=( BOUNDED_CURVE ( )  B_SPLINE_CURVE ( 2, ( #7861, #4917, #1653, #3945, #2643, #2707, #5642 ),
 .UNSPECIFIED., .F., .F. ) 
 B_SPLINE_CURVE_WITH_KNOTS ( ( 3, 2, 2, 3 ),
 ( 0.8000000000000002665, 0.8333333333333334814, 0.8666666666666666963, 0.8887752022894196413 ),
 .UNSPECIFIED. ) 
 CURVE ( )  GEOMETRIC_REPRESENTATION_ITEM ( )  RATIONAL_B_SPLINE_CURVE ( ( 0.9999999999999991118, 0.8660254037844395958, 1.000000000000000000, 0.8660254037844387076, 1.000000000000000000, 0.9111405360107296403, 0.9401542295229903257 ) ) 
 REPRESENTATION_ITEM ( '' )  );
#7924=ORIENTED_EDGE ( 'NONE', *, *, #12947, .T. ) ;
#7925=EDGE_CURVE ( 'NONE', #7130, #8420, #12845, .T. ) ;
#7930=CARTESIAN_POINT ( 'NONE',  ( 3.556430356250015024, 90.00000000000000000, 3.903125000614517504 ) ) ;
#7941=ORIENTED_EDGE ( 'NONE', *, *, #10378, .F. ) ;
#7951=CARTESIAN_POINT ( 'NONE',  ( 25.00000000000000355, 2.000000000000000000, -5.750000000000000000 ) ) ;
#7960=ORIENTED_EDGE ( 'NONE', *, *, #6741, .T. ) ;
#7962=CARTESIAN_POINT ( 'NONE',  ( 50.00000000000000000, 0.000000000000000000, -10.00000000000000000 ) ) ;
#7965=CARTESIAN_POINT ( 'NONE',  ( 3.800000000000015365, 90.00000000000000000, 4.100000000000000533 ) ) ;
#7973=EDGE_CURVE ( 'NONE', #9690, #4278, #10955, .T. ) ;
#7982=DIRECTION ( 'NONE',  ( -0.000000000000000000, -0.000000000000000000, -1.000000000000000000 ) ) ;
#7993=CARTESIAN_POINT ( 'NONE',  ( 60.43447243729646345, 111.3420572890634048, 2.688859442485532991 ) ) ;
#8008=CARTESIAN_POINT ( 'NONE',  ( 50.72178482187499071, 117.2309300971526937, 4.203125000614517326 ) ) ;
#8011=DIRECTION ( 'NONE',  ( 1.000000000000000000, 0.000000000000000000, -1.445602896647339656E-17 ) ) ;
#8012=DIRECTION ( 'NONE',  ( -0.000000000000000000, -0.000000000000000000, -1.000000000000000000 ) ) ;
#8015=VECTOR ( 'NONE', #8813, 1000.000000000000000 ) ;
#8016=PLANE ( 'NONE',  #1974 ) ;
#8024=EDGE_LOOP ( 'NONE', ( #9967, #8167, #8960, #5558 ) ) ;
#8028=CARTESIAN_POINT ( 'NONE',  ( 20.00000000000000355, 121.2009999999999934, 1.500000000000000444 ) ) ;
#8033=AXIS2_PLACEMENT_3D ( 'NONE', #9380, #12526, #10624 ) ;
#8045=VECTOR ( 'NONE', #700, 1000.000000000000000 ) ;
#8050=DIRECTION ( 'NONE',  ( -1.000000000000000000, 0.000000000000000000, 0.000000000000000000 ) ) ;
#8053=ORIENTED_EDGE ( 'NONE', *, *, #2569, .F. ) ;
#8056=VERTEX_POINT ( 'NONE', #10622 ) ;
#8065=ORIENTED_EDGE ( 'NONE', *, *, #666, .T. ) ;
#8066=CARTESIAN_POINT ( 'NONE',  ( 35.00000000000000000, 126.3079067962035822, 4.746875000614517504 ) ) ;
#8070=FACE_OUTER_BOUND ( 'NONE', #12240, .T. ) ;
#8073=CARTESIAN_POINT ( 'NONE',  ( 66.44356964374998142, 108.1539533981018053, 3.265625000614516882 ) ) ;
#8078=LINE ( 'NONE', #11136, #11860 ) ;
#8082=DIRECTION ( 'NONE',  ( -0.000000000000000000, -0.000000000000000000, -1.000000000000000000 ) ) ;
#8109=EDGE_CURVE ( 'NONE', #7130, #4396, #4016, .T. ) ;
#8113=FACE_OUTER_BOUND ( 'NONE', #5079, .T. ) ;
#8114=VERTEX_POINT ( 'NONE', #1790 ) ;
#8120=EDGE_LOOP ( 'NONE', ( #6525, #3655 ) ) ;
#8125=CARTESIAN_POINT ( 'NONE',  ( 66.19999999999993179, 71.98667160128364628, 3.500000001229034208 ) ) ;
#8126=CARTESIAN_POINT ( 'NONE',  ( 50.60000000000001563, 62.98000740192552627, 3.012500001229034829 ) ) ;
#8128=PLANE ( 'NONE',  #11046 ) ;
#8131=CARTESIAN_POINT ( 'NONE',  ( 35.00000000000000000, 126.0266567974326222, 4.437500000000000888 ) ) ;
#8132=CARTESIAN_POINT ( 'NONE',  ( 25.00000000000000355, 0.000000000000000000, 7.349999999999996980 ) ) ;
#8134=ORIENTED_EDGE ( 'NONE', *, *, #11408, .F. ) ;
#8140=ORIENTED_EDGE ( 'NONE', *, *, #2025, .T. ) ;
#8142=VECTOR ( 'NONE', #10488, 1000.000000000000000 ) ;
#8167=ORIENTED_EDGE ( 'NONE', *, *, #1929, .T. ) ;
#8170=ORIENTED_EDGE ( 'NONE', *, *, #2943, .F. ) ;
#8176=FACE_OUTER_BOUND ( 'NONE', #8670, .T. ) ;
#8181=DIRECTION ( 'NONE',  ( -0.000000000000000000, -0.000000000000000000, -1.000000000000000000 ) ) ;
#8182=EDGE_CURVE ( 'NONE', #7595, #6209, #9957, .T. ) ;
#8185=( BOUNDED_CURVE ( )  B_SPLINE_CURVE ( 2, ( #2999, #5078, #12151, #10967, #9071, #1152, #7246 ),
 .UNSPECIFIED., .F., .F. ) 
 B_SPLINE_CURVE_WITH_KNOTS ( ( 3, 2, 2, 3 ),
 ( 0.1999999999999999833, 0.2333333333333333925, 0.2666666666666668295, 0.3000000000000002109 ),
 .UNSPECIFIED. ) 
 CURVE ( )  GEOMETRIC_REPRESENTATION_ITEM ( )  RATIONAL_B_SPLINE_CURVE ( ( 1.000000000000000222, 0.8660254037844385966, 1.000000000000000000, 0.8660254037844387076, 1.000000000000000000, 0.8660254037844378194, 1.000000000000000888 ) ) 
 REPRESENTATION_ITEM ( '' )  );
#8189=CARTESIAN_POINT ( 'NONE',  ( 66.20000000000000284, 71.98667160128370313, 3.050000001229034474 ) ) ;
#8192=EDGE_LOOP ( 'NONE', ( #6289, #9552, #4663, #2881 ) ) ;
#8193=CARTESIAN_POINT ( 'NONE',  ( 35.00000000000000000, 126.0266567974326222, 3.537500000000000089 ) ) ;
#8195=ORIENTED_EDGE ( 'NONE', *, *, #4002, .T. ) ;
#8196=DIRECTION ( 'NONE',  ( 1.000000000000000000, 0.000000000000000000, 2.891205793294678696E-17 ) ) ;
#8197=ORIENTED_EDGE ( 'NONE', *, *, #11930, .T. ) ;
#8198=CARTESIAN_POINT ( 'NONE',  ( 35.00000000000000000, 90.00000000000000000, 5.000000000000000000 ) ) ;
#8203=CARTESIAN_POINT ( 'NONE',  ( 66.44356964374999563, 71.84604660189820891, 3.640625000614517326 ) ) ;
#8205=CARTESIAN_POINT ( 'NONE',  ( 3.556430356250015024, 90.00000000000000000, 3.059375000614517059 ) ) ;
#8218=ORIENTED_EDGE ( 'NONE', *, *, #1382, .F. ) ;
#8222=ADVANCED_FACE ( 'NONE', ( #2905 ), #10593, .F. ) ;
#8228=ORIENTED_EDGE ( 'NONE', *, *, #9782, .T. ) ;
#8233=ADVANCED_FACE ( 'NONE', ( #12374 ), #450, .F. ) ;
#8235=CARTESIAN_POINT ( 'NONE',  ( 19.40000000000000924, 117.0199925980744666, 2.787500001229034297 ) ) ;
#8239=VECTOR ( 'NONE', #4814, 1000.000000000000000 ) ;
#8242=FACE_BOUND ( 'NONE', #1287, .T. ) ;
#8243=ORIENTED_EDGE ( 'NONE', *, *, #6771, .T. ) ;
#8255=CARTESIAN_POINT ( 'NONE',  ( 66.19999999999998863, 90.00000000000000000, 3.537500001229034297 ) ) ;
#8258=EDGE_CURVE ( 'NONE', #10818, #12910, #11925, .T. ) ;
#8260=CARTESIAN_POINT ( 'NONE',  ( 66.20000000000000284, 71.98667160128370313, 4.737500000000000711 ) ) ;
#8269=CARTESIAN_POINT ( 'NONE',  ( 50.72178482187499071, 117.2309300971526937, 2.853125000614517237 ) ) ;
#8270=CARTESIAN_POINT ( 'NONE',  ( 66.44356964374999563, 90.00000000000000000, 4.634375000614516793 ) ) ;
#8277=DIRECTION ( 'NONE',  ( -0.000000000000000000, -0.000000000000000000, -1.000000000000000000 ) ) ;
#8296=DIRECTION ( 'NONE',  ( -1.000000000000000000, 0.000000000000000000, -0.000000000000000000 ) ) ;
#8297=EDGE_LOOP ( 'NONE', ( #9106, #12647, #8134, #8635, #8548, #4699, #10062, #11298 ) ) ;
#8307=ORIENTED_EDGE ( 'NONE', *, *, #11838, .T. ) ;
#8308=AXIS2_PLACEMENT_3D ( 'NONE', #10820, #10944, #10755 ) ;
#8323=CARTESIAN_POINT ( 'NONE',  ( 66.19999999999998863, 90.00000000000000000, 3.875000000000000000 ) ) ;
#8335=CARTESIAN_POINT ( 'NONE',  ( 19.27821517812503060, 62.76906990284727783, 4.484375000614516438 ) ) ;
#8337=DIRECTION ( 'NONE',  ( 1.000000000000000000, 0.000000000000000000, 0.000000000000000000 ) ) ;
#8360=CARTESIAN_POINT ( 'NONE',  ( 19.27821517812500574, 117.2309300971526937, 4.728125000614516793 ) ) ;
#8371=VERTEX_POINT ( 'NONE', #9941 ) ;
#8376=VERTEX_POINT ( 'NONE', #12640 ) ;
#8384=CIRCLE ( 'NONE', #7545, 1.500000000000001332 ) ;
#8391=CARTESIAN_POINT ( 'NONE',  ( 66.19999999999988916, 71.98667160128361786, 4.400000001229033231 ) ) ;
#8399=CARTESIAN_POINT ( 'NONE',  ( 35.00000000000000000, 126.3079067962036106, 4.296875000614517326 ) ) ;
#8400=EDGE_CURVE ( 'NONE', #4218, #6538, #7662, .T. ) ;
#8401=DIRECTION ( 'NONE',  ( -0.000000000000000000, -0.000000000000000000, -1.000000000000000000 ) ) ;
#8418=ADVANCED_FACE ( 'NONE', ( #6931, #42, #8242, #3146 ), #4126, .T. ) ;
#8420=VERTEX_POINT ( 'NONE', #3213 ) ;
#8427=CARTESIAN_POINT ( 'NONE',  ( 50.00000000000000000, 2.000000000000000000, 10.00000000000000000 ) ) ;
#8429=VECTOR ( 'NONE', #5864, 1000.000000000000000 ) ;
#8432=ORIENTED_EDGE ( 'NONE', *, *, #9603, .T. ) ;
#8441=ORIENTED_EDGE ( 'NONE', *, *, #9657, .F. ) ;
#8453=CARTESIAN_POINT ( 'NONE',  ( 3.556430356250014579, 108.1539533981018053, 3.471875000614516704 ) ) ;
#8462=CARTESIAN_POINT ( 'NONE',  ( 35.00000000000000000, 90.00000000000000000, 5.000000000000000000 ) ) ;
#8464=CARTESIAN_POINT ( 'NONE',  ( 3.556430356250028790, 71.84604660189818048, 4.446875000614517681 ) ) ;
#8466=ADVANCED_FACE ( 'NONE', ( #8113 ), #2297, .F. ) ;
#8479=STYLED_ITEM('',(#13016),#3242);
#8482=VERTEX_POINT ( 'NONE', #7126 ) ;
#8484=CARTESIAN_POINT ( 'NONE',  ( 30.00000000000000711, 0.000000000000000000, 10.00000000000000000 ) ) ;
#8491=CARTESIAN_POINT ( 'NONE',  ( 35.00000000000000711, 53.69209320379639649, 4.465625000614517504 ) ) ;
#8502=ORIENTED_EDGE ( 'NONE', *, *, #200, .T. ) ;
#8514=EDGE_CURVE ( 'NONE', #1636, #10706, #3046, .T. ) ;
#8521=CARTESIAN_POINT ( 'NONE',  ( 66.19999999999988916, 71.98667160128361786, 3.050000001229034030 ) ) ;
#8526=ADVANCED_FACE ( 'NONE', ( #8176 ), #11177, .F. ) ;
#8532=CARTESIAN_POINT ( 'NONE',  ( 3.556430356250014579, 108.1539533981018053, 4.315625000614517148 ) ) ;
#8534=CARTESIAN_POINT ( 'NONE',  ( 4.800000000000015810, 90.00000000000000000, 5.000000000000000000 ) ) ;
#8535=CARTESIAN_POINT ( 'NONE',  ( 49.99999999999996447, 90.00000000000000000, -5.000000000000000000 ) ) ;
#8548=ORIENTED_EDGE ( 'NONE', *, *, #6843, .F. ) ;
#8554=ORIENTED_EDGE ( 'NONE', *, *, #10833, .F. ) ;
#8555=LINE ( 'NONE', #12545, #10764 ) ;
#8560=CARTESIAN_POINT ( 'NONE',  ( 22.99999999999998579, 90.00000000000000000, -5.000000000000000000 ) ) ;
#8563=DIRECTION ( 'NONE',  ( -0.000000000000000000, -0.000000000000000000, -1.000000000000000000 ) ) ;
#8572=VECTOR ( 'NONE', #8884, 1000.000000000000000 ) ;
#8575=FACE_OUTER_BOUND ( 'NONE', #7313, .T. ) ;
#8586=CARTESIAN_POINT ( 'NONE',  ( 3.556430356250015024, 90.00000000000000000, 3.959375000614517415 ) ) ;
#8587=EDGE_LOOP ( 'NONE', ( #9734, #8195, #3189 ) ) ;
#8601=ADVANCED_FACE ( 'NONE', ( #3472 ), #11569, .F. ) ;
#8613=DIRECTION ( 'NONE',  ( -0.000000000000000000, -0.000000000000000000, -1.000000000000000000 ) ) ;
#8614=ORIENTED_EDGE ( 'NONE', *, *, #5011, .F. ) ;
#8616=CARTESIAN_POINT ( 'NONE',  ( 50.72178482187499071, 117.2309300971526937, 4.203125000614517326 ) ) ;
#8617=VERTEX_POINT ( 'NONE', #11370 ) ;
#8620=ORIENTED_EDGE ( 'NONE', *, *, #9902, .F. ) ;
#8635=ORIENTED_EDGE ( 'NONE', *, *, #11951, .F. ) ;
#8638=EDGE_LOOP ( 'NONE', ( #802, #6155, #9150, #10658 ) ) ;
#8645=EDGE_CURVE ( 'NONE', #11848, #8056, #1364, .T. ) ;
#8650=ORIENTED_EDGE ( 'NONE', *, *, #11181, .F. ) ;
#8652=ORIENTED_EDGE ( 'NONE', *, *, #1437, .T. ) ;
#8653=DIRECTION ( 'NONE',  ( 0.000000000000000000, 1.000000000000000000, 0.000000000000000000 ) ) ;
#8655=LINE ( 'NONE', #11658, #5789 ) ;
#8656=CARTESIAN_POINT ( 'NONE',  ( 3.556430356250014579, 108.1539533981018053, 3.865625000614517415 ) ) ;
#8660=CARTESIAN_POINT ( 'NONE',  ( 50.60000000000001563, 62.98000740192552627, 3.912500001229034297 ) ) ;
#8666=CARTESIAN_POINT ( 'NONE',  ( 66.44356964374998142, 108.1539533981018053, 4.221875000614517148 ) ) ;
#8667=ORIENTED_EDGE ( 'NONE', *, *, #10848, .F. ) ;
#8669=CARTESIAN_POINT ( 'NONE',  ( 3.800000000000015365, 90.00000000000000000, 5.000000000000000000 ) ) ;
#8670=EDGE_LOOP ( 'NONE', ( #9596, #1060, #2442, #12686 ) ) ;
#8675=FACE_OUTER_BOUND ( 'NONE', #6122, .T. ) ;
#8679=CARTESIAN_POINT ( 'NONE',  ( 3.556430356250015024, 90.00000000000000000, 3.003125000614517148 ) ) ;
#8683=EDGE_LOOP ( 'NONE', ( #8243, #6535 ) ) ;
#8689=CYLINDRICAL_SURFACE ( 'NONE', #7912, 31.19999999999998863 ) ;
#8690=AXIS2_PLACEMENT_3D ( 'NONE', #2268, #7096, #144 ) ;
#8696=CARTESIAN_POINT ( 'NONE',  ( 25.00000000000000355, 2.000000000000000000, -4.150000000000007461 ) ) ;
#8697=CARTESIAN_POINT ( 'NONE',  ( 17.66025403784438197, 77.14656965084323303, -1.000000000000000000 ) ) ;
#8718=CARTESIAN_POINT ( 'NONE',  ( 66.44356964374999563, 71.84604660189820891, 3.640625000614517326 ) ) ;
#8719=LINE ( 'NONE', #3948, #810 ) ;
#8721=ADVANCED_FACE ( 'NONE', ( #7581 ), #5480, .T. ) ;
#8727=DIRECTION ( 'NONE',  ( -0.000000000000000000, 1.000000000000000000, -0.000000000000000000 ) ) ;
#8728=CARTESIAN_POINT ( 'NONE',  ( 3.556430356250014579, 108.1539533981018053, 3.021875000614517415 ) ) ;
#8739=CARTESIAN_POINT ( 'NONE',  ( 50.72178482187499071, 117.2309300971526937, 3.303125000614517415 ) ) ;
#8745=EDGE_LOOP ( 'NONE', ( #1903, #10085, #178, #8849 ) ) ;
#8754=( BOUNDED_CURVE ( )  B_SPLINE_CURVE ( 2, ( #3490, #8521, #2701, #7470, #12510, #11455, #7664 ),
 .UNSPECIFIED., .F., .F. ) 
 B_SPLINE_CURVE_WITH_KNOTS ( ( 3, 2, 2, 3 ),
 ( 0.7000000000000001776, 0.7333333333333335036, 0.7666666666666669405, 0.8000000000000002665 ),
 .UNSPECIFIED. ) 
 CURVE ( )  GEOMETRIC_REPRESENTATION_ITEM ( )  RATIONAL_B_SPLINE_CURVE ( ( 0.9999999999999991118, 0.8660254037844395958, 1.000000000000000000, 0.8660254037844387076, 1.000000000000000000, 0.8660254037844378194, 1.000000000000000888 ) ) 
 REPRESENTATION_ITEM ( '' )  );
#8755=CARTESIAN_POINT ( 'NONE',  ( 35.00000000000000000, 90.00000000000000000, 1.500000000000000888 ) ) ;
#8761=EDGE_LOOP ( 'NONE', ( #12582, #2609, #346, #10667 ) ) ;
#8763=ORIENTED_EDGE ( 'NONE', *, *, #12712, .F. ) ;
#8781=CARTESIAN_POINT ( 'NONE',  ( 50.72178482187499071, 117.2309300971526937, 3.753125000614517592 ) ) ;
#8787=CARTESIAN_POINT ( 'NONE',  ( 50.00000000000000000, 62.64236852357281293, 5.000000000000000000 ) ) ;
#8797=CARTESIAN_POINT ( 'NONE',  ( 21.49999999999998579, 90.00000000000000000, -8.000000000000000000 ) ) ;
#8802=CARTESIAN_POINT ( 'NONE',  ( 64.31840976852106451, 100.6710284717588024, 2.999476386674974737 ) ) ;
#8803=CARTESIAN_POINT ( 'NONE',  ( 50.72178482187499071, 117.2309300971526937, 3.753125000614517592 ) ) ;
#8807=DIRECTION ( 'NONE',  ( 0.000000000000000000, 0.000000000000000000, -1.000000000000000000 ) ) ;
#8811=EDGE_CURVE ( 'NONE', #9386, #10351, #2874, .T. ) ;
#8813=DIRECTION ( 'NONE',  ( 0.000000000000000000, 0.000000000000000000, -1.000000000000000000 ) ) ;
#8837=DIRECTION ( 'NONE',  ( -1.000000000000000000, 0.000000000000000000, 0.000000000000000000 ) ) ;
#8839=EDGE_CURVE ( 'NONE', #2101, #12533, #10665, .T. ) ;
#8841=CARTESIAN_POINT ( 'NONE',  ( 19.27821517812500574, 117.2309300971526937, 4.278125000614516615 ) ) ;
#8844=DIRECTION ( 'NONE',  ( -0.000000000000000000, -1.000000000000000000, -0.000000000000000000 ) ) ;
#8847=LINE ( 'NONE', #8787, #2709 ) ;
#8849=ORIENTED_EDGE ( 'NONE', *, *, #2532, .F. ) ;
#8852=EDGE_LOOP ( 'NONE', ( #1226, #3681, #2558, #10550, #11165, #7502, #10009, #10451 ) ) ;
#8854=CARTESIAN_POINT ( 'NONE',  ( 66.44356964374999563, 71.84604660189820891, 4.146875000614517859 ) ) ;
#8855=ORIENTED_EDGE ( 'NONE', *, *, #11067, .F. ) ;
#8859=CARTESIAN_POINT ( 'NONE',  ( 45.00000000000000000, 2.000000000000000000, 5.750000000000000888 ) ) ;
#8876=LINE ( 'NONE', #5013, #7168 ) ;
#8884=DIRECTION ( 'NONE',  ( -0.000000000000000000, -0.000000000000000000, -1.000000000000000000 ) ) ;
#8906=CARTESIAN_POINT ( 'NONE',  ( 66.44356964374998142, 108.1539533981018053, 3.715625000614517948 ) ) ;
#8910=EDGE_CURVE ( 'NONE', #8371, #12624, #4350, .T. ) ;
#8923=DIRECTION ( 'NONE',  ( -1.000000000000000000, 0.000000000000000000, 0.000000000000000000 ) ) ;
#8924=AXIS2_PLACEMENT_3D ( 'NONE', #8797, #933, #8923 ) ;
#8932=AXIS2_PLACEMENT_3D ( 'NONE', #11449, #4456, #2437 ) ;
#8935=CARTESIAN_POINT ( 'NONE',  ( 50.00000000000000000, 0.000000000000000000, -10.00000000000000000 ) ) ;
#8939=CARTESIAN_POINT ( 'NONE',  ( 45.00000000000000000, 2.000000000000000000, -7.349999999999993427 ) ) ;
#8946=ORIENTED_EDGE ( 'NONE', *, *, #12642, .F. ) ;
#8960=ORIENTED_EDGE ( 'NONE', *, *, #2802, .T. ) ;
#8962=ORIENTED_EDGE ( 'NONE', *, *, #6268, .F. ) ;
#8965=CARTESIAN_POINT ( 'NONE',  ( 35.00000000000000711, 53.97334320256736362, 3.425000001229034474 ) ) ;
#8967=CARTESIAN_POINT ( 'NONE',  ( 3.800000000000015365, 108.0133283987163111, 3.725000001229034297 ) ) ;
#8979=CARTESIAN_POINT ( 'NONE',  ( 3.556430356250028790, 71.84604660189818048, 3.490625000614517415 ) ) ;
#8983=CARTESIAN_POINT ( 'NONE',  ( 20.00000000000000355, 2.000000000000001776, -1.499999999999999556 ) ) ;
#8996=ADVANCED_FACE ( 'NONE', ( #12329 ), #3378, .F. ) ;
#8997=CARTESIAN_POINT ( 'NONE',  ( 0.000000000000000000, 0.000000000000000000, 0.000000000000000000 ) ) ;
#9001=LINE ( 'NONE', #8939, #11774 ) ;
#9002=EDGE_LOOP ( 'NONE', ( #12897, #10912 ) ) ;
#9010=CARTESIAN_POINT ( 'NONE',  ( 40.00000000000000000, 0.000000000000000000, 10.00000000000000000 ) ) ;
#9020=CARTESIAN_POINT ( 'NONE',  ( 45.00000000000000000, 2.000000000000001332, 5.750000000000000888 ) ) ;
#9025=ORIENTED_EDGE ( 'NONE', *, *, #3108, .F. ) ;
#9026=CARTESIAN_POINT ( 'NONE',  ( 46.99999999999995737, 90.00000000000000000, -8.000000000000000000 ) ) ;
#9031=CARTESIAN_POINT ( 'NONE',  ( 3.800000000000015365, 90.00000000000000000, 3.762500001229034385 ) ) ;
#9035=CARTESIAN_POINT ( 'NONE',  ( 66.20000000000000284, 71.98667160128370313, 4.287500000000000533 ) ) ;
#9041=LINE ( 'NONE', #4277, #2583 ) ;
#9044=CARTESIAN_POINT ( 'NONE',  ( 66.44356964374999563, 90.00000000000000000, 3.678125000614516971 ) ) ;
#9049=CARTESIAN_POINT ( 'NONE',  ( 35.00000000000000000, 90.00000000000000000, 5.000000000000000000 ) ) ;
#9051=CARTESIAN_POINT ( 'NONE',  ( 17.66025403784438197, 77.14656965084323303, 1.000000000000000000 ) ) ;
#9066=DIRECTION ( 'NONE',  ( -0.000000000000000000, 1.000000000000000000, -0.000000000000000000 ) ) ;
#9069=AXIS2_PLACEMENT_3D ( 'NONE', #3518, #8613, #7501 ) ;
#9071=CARTESIAN_POINT ( 'NONE',  ( 50.59999999999999432, 117.0199925980744666, 4.062500001229034652 ) ) ;
#9072=EDGE_CURVE ( 'NONE', #7376, #2423, #9701, .T. ) ;
#9077=ORIENTED_EDGE ( 'NONE', *, *, #2858, .F. ) ;
#9080=VECTOR ( 'NONE', #6723, 1000.000000000000000 ) ;
#9081=EDGE_LOOP ( 'NONE', ( #9025, #930, #4339, #2705 ) ) ;
#9100=DIRECTION ( 'NONE',  ( 1.000000000000000000, 0.000000000000000000, -0.000000000000000000 ) ) ;
#9103=CARTESIAN_POINT ( 'NONE',  ( 19.27821517812500574, 117.2309300971526937, 4.334375000614516971 ) ) ;
#9106=ORIENTED_EDGE ( 'NONE', *, *, #9963, .F. ) ;
#9107=DIRECTION ( 'NONE',  ( 0.000000000000000000, 0.000000000000000000, 1.000000000000000000 ) ) ;
#9108=VERTEX_POINT ( 'NONE', #11605 ) ;
#9110=CARTESIAN_POINT ( 'NONE',  ( 19.27821517812500574, 117.2309300971526937, 3.378125000614517148 ) ) ;
#9122=LINE ( 'NONE', #7293, #2634 ) ;
#9141=ORIENTED_EDGE ( 'NONE', *, *, #3130, .F. ) ;
#9145=VERTEX_POINT ( 'NONE', #9640 ) ;
#9150=ORIENTED_EDGE ( 'NONE', *, *, #12108, .T. ) ;
#9161=( NAMED_UNIT ( * ) SI_UNIT ( $, .STERADIAN. ) SOLID_ANGLE_UNIT ( ) );
#9163=DIRECTION ( 'NONE',  ( -0.8660254037844365982, -0.5000000000000036637, 0.000000000000000000 ) ) ;
#9166=CARTESIAN_POINT ( 'NONE',  ( 35.00000000000000711, 53.97334320256736362, 3.312500000000000000 ) ) ;
#9170=DIRECTION ( 'NONE',  ( -0.000000000000000000, -0.000000000000000000, -1.000000000000000000 ) ) ;
#9173=DIRECTION ( 'NONE',  ( -0.000000000000000000, -1.000000000000000000, -0.000000000000000000 ) ) ;
#9175=CARTESIAN_POINT ( 'NONE',  ( 19.27821517812500574, 117.2309300971526937, 3.828125000614516882 ) ) ;
#9182=AXIS2_PLACEMENT_3D ( 'NONE', #2115, #7143, #11125 ) ;
#9192=CIRCLE ( 'NONE', #2095, 1.599999999999997202 ) ;
#9212=EDGE_LOOP ( 'NONE', ( #1771, #4260, #5934, #7326 ) ) ;
#9223=ORIENTED_EDGE ( 'NONE', *, *, #2943, .T. ) ;
#9226=EDGE_CURVE ( 'NONE', #12533, #5692, #8847, .T. ) ;
#9232=CARTESIAN_POINT ( 'NONE',  ( 66.44356964374999563, 90.00000000000000000, 4.634375000614516793 ) ) ;
#9236=CARTESIAN_POINT ( 'NONE',  ( 45.00000000000000000, 2.000000000000000000, -5.750000000000000000 ) ) ;
#9240=CARTESIAN_POINT ( 'NONE',  ( 0.000000000000000000, 0.000000000000000000, 10.00000000000000000 ) ) ;
#9241=CARTESIAN_POINT ( 'NONE',  ( 3.556430356250014579, 108.1539533981018053, 2.965625000614517504 ) ) ;
#9243=CARTESIAN_POINT ( 'NONE',  ( 3.556430356250014579, 108.1539533981018053, 3.921875000614517326 ) ) ;
#9246=AXIS2_PLACEMENT_3D ( 'NONE', #9487, #1574, #9747 ) ;
#9254=FACE_OUTER_BOUND ( 'NONE', #8297, .T. ) ;
#9255=EDGE_LOOP ( 'NONE', ( #9587, #11698, #10105, #8962 ) ) ;
#9256=VECTOR ( 'NONE', #3978, 1000.000000000000000 ) ;
#9266=COLOUR_RGB ( '',0.8941176470588234615, 0.8941176470588234615, 0.8941176470588234615 ) ;
#9284=ORIENTED_EDGE ( 'NONE', *, *, #11078, .T. ) ;
#9291=ORIENTED_EDGE ( 'NONE', *, *, #2481, .F. ) ;
#9293=VECTOR ( 'NONE', #9611, 1000.000000000000000 ) ;
#9295=CARTESIAN_POINT ( 'NONE',  ( 19.40000000000000924, 117.0199925980744666, 3.237500001229034030 ) ) ;
#9296=CARTESIAN_POINT ( 'NONE',  ( 40.00000000000000000, 90.00000000000000000, -8.000000000000000000 ) ) ;
#9299=CARTESIAN_POINT ( 'NONE',  ( 66.19999999999998863, 90.00000000000000000, 3.425000000000000266 ) ) ;
#9311=DIRECTION ( 'NONE',  ( 0.000000000000000000, 0.000000000000000000, 1.000000000000000000 ) ) ;
#9312=AXIS2_PLACEMENT_3D ( 'NONE', #10950, #11876, #875 ) ;
#9320=LINE ( 'NONE', #11279, #4276 ) ;
#9339=VERTEX_POINT ( 'NONE', #6157 ) ;
#9342=CARTESIAN_POINT ( 'NONE',  ( 3.800000000000015365, 90.00000000000000000, 2.862500001229034474 ) ) ;
#9353=ORIENTED_EDGE ( 'NONE', *, *, #200, .F. ) ;
#9363=DIRECTION ( 'NONE',  ( -0.9396926073018736503, -0.3420201803727477285, 0.000000000000000000 ) ) ;
#9367=VECTOR ( 'NONE', #11496, 1000.000000000000000 ) ;
#9376=AXIS2_PLACEMENT_3D ( 'NONE', #4222, #12193, #8337 ) ;
#9377=CARTESIAN_POINT ( 'NONE',  ( 35.00000000000000000, 90.00000000000000000, -5.000000000000000000 ) ) ;
#9378=CARTESIAN_POINT ( 'NONE',  ( 25.00000000000000355, 2.000000000000001332, -5.750000000000000000 ) ) ;
#9380=CARTESIAN_POINT ( 'NONE',  ( 48.49999999999995737, 90.00000000000000000, -8.000000000000000000 ) ) ;
#9386=VERTEX_POINT ( 'NONE', #8132 ) ;
#9387=DIRECTION ( 'NONE',  ( -0.000000000000000000, -0.000000000000000000, -1.000000000000000000 ) ) ;
#9388=DIRECTION ( 'NONE',  ( -0.000000000000000000, -0.000000000000000000, -1.000000000000000000 ) ) ;
#9392=CARTESIAN_POINT ( 'NONE',  ( 35.00000000000000000, 90.00000000000000000, -5.000000000000000000 ) ) ;
#9393=DIRECTION ( 'NONE',  ( 1.000000000000000000, 0.000000000000000000, -0.000000000000000000 ) ) ;
#9414=CARTESIAN_POINT ( 'NONE',  ( 3.799999999999904787, 71.98667160128373155, 3.237499999999999822 ) ) ;
#9433=PLANE ( 'NONE',  #7329 ) ;
#9434=EDGE_CURVE ( 'NONE', #5827, #8056, #2315, .T. ) ;
#9435=PLANE ( 'NONE',  #5780 ) ;
#9436=CARTESIAN_POINT ( 'NONE',  ( 35.00000000000000711, 53.69209320379639649, 4.521875000614516971 ) ) ;
#9438=CARTESIAN_POINT ( 'NONE',  ( 50.72178482187499071, 117.2309300971526937, 4.653125000614517504 ) ) ;
#9440=( BOUNDED_CURVE ( )  B_SPLINE_CURVE ( 2, ( #11448, #11384, #3291, #3415, #7205, #3355, #1308 ),
 .UNSPECIFIED., .F., .F. ) 
 B_SPLINE_CURVE_WITH_KNOTS ( ( 3, 2, 2, 3 ),
 ( 0.1000000000000001860, 0.1333333333333334425, 0.1666666666666666852, 0.2000000000000000111 ),
 .UNSPECIFIED. ) 
 CURVE ( )  GEOMETRIC_REPRESENTATION_ITEM ( )  RATIONAL_B_SPLINE_CURVE ( ( 0.9999999999999992228, 0.8660254037844394848, 1.000000000000000000, 0.8660254037844387076, 1.000000000000000000, 0.8660254037844388186, 0.9999999999999998890 ) ) 
 REPRESENTATION_ITEM ( '' )  );
#9448=CARTESIAN_POINT ( 'NONE',  ( 3.800000000000015810, 108.0133283987162969, 4.962499999999999467 ) ) ;
#9453=ORIENTED_EDGE ( 'NONE', *, *, #10848, .T. ) ;
#9455=PLANE ( 'NONE',  #5930 ) ;
#9457=FACE_BOUND ( 'NONE', #7700, .T. ) ;
#9461=CARTESIAN_POINT ( 'NONE',  ( 66.44356964374999563, 90.00000000000000000, 4.578125000614516438 ) ) ;
#9462=VERTEX_POINT ( 'NONE', #327 ) ;
#9468=VECTOR ( 'NONE', #10961, 1000.000000000000000 ) ;
#9475=CARTESIAN_POINT ( 'NONE',  ( 35.00000000000000000, 90.00000000000000000, 5.000000000000000000 ) ) ;
#9479=EDGE_CURVE ( 'NONE', #10380, #4511, #3345, .T. ) ;
#9481=ORIENTED_EDGE ( 'NONE', *, *, #6361, .F. ) ;
#9484=EDGE_CURVE ( 'NONE', #5315, #1634, #7041, .T. ) ;
#9487=CARTESIAN_POINT ( 'NONE',  ( 45.00000000000000000, 2.000000000000001332, -5.750000000000000000 ) ) ;
#9495=CARTESIAN_POINT ( 'NONE',  ( 66.44356964374998142, 108.1539533981018053, 3.321875000614517237 ) ) ;
#9496=ORIENTED_EDGE ( 'NONE', *, *, #11511, .F. ) ;
#9497=DIRECTION ( 'NONE',  ( -1.000000000000000000, -0.000000000000000000, -0.000000000000000000 ) ) ;
#9502=ORIENTED_EDGE ( 'NONE', *, *, #8910, .F. ) ;
#9503=DIRECTION ( 'NONE',  ( 0.000000000000000000, 0.000000000000000000, 1.000000000000000000 ) ) ;
#9505=FACE_OUTER_BOUND ( 'NONE', #10206, .T. ) ;
#9507=CYLINDRICAL_SURFACE ( 'NONE', #12925, 1.599999999999992095 ) ;
#9519=ADVANCED_FACE ( 'NONE', ( #11391, #6612 ), #389, .F. ) ;
#9526=LINE ( 'NONE', #8484, #10738 ) ;
#9531=ORIENTED_EDGE ( 'NONE', *, *, #2605, .T. ) ;
#9532=FACE_OUTER_BOUND ( 'NONE', #9255, .T. ) ;
#9543=EDGE_CURVE ( 'NONE', #11641, #4459, #6546, .T. ) ;
#9550=CARTESIAN_POINT ( 'NONE',  ( 19.40000000000002700, 62.98000740192551206, 3.275000000000000355 ) ) ;
#9552=ORIENTED_EDGE ( 'NONE', *, *, #739, .F. ) ;
#9559=ADVANCED_FACE ( 'NONE', ( #7599 ), #588, .F. ) ;
#9568=FACE_OUTER_BOUND ( 'NONE', #3716, .T. ) ;
#9581=CARTESIAN_POINT ( 'NONE',  ( 66.19999999999998863, 90.00000000000000000, 5.000000000000000000 ) ) ;
#9587=ORIENTED_EDGE ( 'NONE', *, *, #666, .F. ) ;
#9593=ORIENTED_EDGE ( 'NONE', *, *, #2993, .T. ) ;
#9595=CARTESIAN_POINT ( 'NONE',  ( 50.72178482187501203, 62.76906990284730625, 3.153125000614517504 ) ) ;
#9596=ORIENTED_EDGE ( 'NONE', *, *, #6031, .F. ) ;
#9601=CARTESIAN_POINT ( 'NONE',  ( 66.19999999999998863, 90.00000000000000000, 5.000000000000000000 ) ) ;
#9603=EDGE_CURVE ( 'NONE', #5282, #4450, #8754, .T. ) ;
#9609=CARTESIAN_POINT ( 'NONE',  ( 25.00000000000000355, 2.000000000000000000, 7.349999999999991651 ) ) ;
#9611=DIRECTION ( 'NONE',  ( -0.000000000000000000, -0.000000000000000000, -1.000000000000000000 ) ) ;
#9619=ORIENTED_EDGE ( 'NONE', *, *, #9434, .F. ) ;
#9624=ORIENTED_EDGE ( 'NONE', *, *, #11067, .T. ) ;
#9625=CARTESIAN_POINT ( 'NONE',  ( 66.44356964374999563, 71.84604660189820891, 4.146875000614517859 ) ) ;
#9633=PLANE ( 'NONE',  #6287 ) ;
#9635=CARTESIAN_POINT ( 'NONE',  ( 3.556430356250014579, 108.1539533981018053, 4.765625000614517326 ) ) ;
#9637=DIRECTION ( 'NONE',  ( 0.000000000000000000, 0.000000000000000000, -1.000000000000000000 ) ) ;
#9640=CARTESIAN_POINT ( 'NONE',  ( 25.00000000000000355, 0.000000000000000000, 4.150000000000003020 ) ) ;
#9656=CARTESIAN_POINT ( 'NONE',  ( 19.27821517812503060, 62.76906990284727783, 3.978125000614516793 ) ) ;
#9657=EDGE_CURVE ( 'NONE', #9462, #716, #12942, .T. ) ;
#9658=CARTESIAN_POINT ( 'NONE',  ( 25.00000000000000355, 0.000000000000000000, -4.150000000000003020 ) ) ;
#9659=CARTESIAN_POINT ( 'NONE',  ( 30.00000000000000711, 0.000000000000000000, -10.00000000000000000 ) ) ;
#9669=DIRECTION ( 'NONE',  ( -1.000000000000000000, 0.000000000000000000, -2.780005570475653612E-17 ) ) ;
#9681=CARTESIAN_POINT ( 'NONE',  ( 21.49999999999998579, 90.00000000000000000, -5.000000000000000000 ) ) ;
#9690=VERTEX_POINT ( 'NONE', #6738 ) ;
#9695=CARTESIAN_POINT ( 'NONE',  ( 3.800000000000015365, 90.00000000000000000, 4.662500001229034297 ) ) ;
#9697=CARTESIAN_POINT ( 'NONE',  ( 35.00000000000000000, 90.00000000000000000, 5.000000000000000000 ) ) ;
#9699=CARTESIAN_POINT ( 'NONE',  ( 3.800000000000015365, 90.00000000000000000, 5.000000000000000000 ) ) ;
#9701=LINE ( 'NONE', #11535, #807 ) ;
#9705=CARTESIAN_POINT ( 'NONE',  ( 3.556430356250028790, 71.84604660189818048, 3.096875000614517592 ) ) ;
#9708=ADVANCED_FACE ( 'NONE', ( #11715, #11845, #2952, #12766, #5884 ), #7787, .T. ) ;
#9710=EDGE_LOOP ( 'NONE', ( #1346, #9742, #12076, #2425, #7209, #3236, #6925, #11500, #8228, #3997, #7252, #2747 ) ) ;
#9711=AXIS2_PLACEMENT_3D ( 'NONE', #5745, #3729, #7712 ) ;
#9713=AXIS2_PLACEMENT_3D ( 'NONE', #9378, #10561, #5648 ) ;
#9716=LINE ( 'NONE', #1739, #8239 ) ;
#9717=VECTOR ( 'NONE', #2876, 1000.000000000000000 ) ;
#9719=CARTESIAN_POINT ( 'NONE',  ( 66.44356964374998142, 108.1539533981018053, 4.165625000614516793 ) ) ;
#9720=VECTOR ( 'NONE', #2950, 1000.000000000000000 ) ;
#9724=CYLINDRICAL_SURFACE ( 'NONE', #5576, 31.19999999999998863 ) ;
#9729=AXIS2_PLACEMENT_3D ( 'NONE', #472, #404, #11668 ) ;
#9734=ORIENTED_EDGE ( 'NONE', *, *, #2982, .F. ) ;
#9737=CARTESIAN_POINT ( 'NONE',  ( 3.800000000000015365, 90.00000000000000000, 5.000000000000000000 ) ) ;
#9742=ORIENTED_EDGE ( 'NONE', *, *, #10607, .T. ) ;
#9747=DIRECTION ( 'NONE',  ( 0.000000000000000000, 0.000000000000000000, 1.000000000000000000 ) ) ;
#9750=AXIS2_PLACEMENT_3D ( 'NONE', #9976, #5859, #1008 ) ;
#9763=CARTESIAN_POINT ( 'NONE',  ( 19.27821517812500574, 117.2309300971526937, 2.928125000614517415 ) ) ;
#9772=CARTESIAN_POINT ( 'NONE',  ( 60.63303222545420823, 111.5086687406912347, 2.885734441871016021 ) ) ;
#9779=SURFACE_SIDE_STYLE ('',( #1736 ) ) ;
#9782=EDGE_CURVE ( 'NONE', #10175, #1050, #1915, .T. ) ;
#9784=CARTESIAN_POINT ( 'NONE',  ( 35.00000000000000711, 53.69209320379639649, 4.015625000614517326 ) ) ;
#9789=ORIENTED_EDGE ( 'NONE', *, *, #1841, .F. ) ;
#9790=FACE_BOUND ( 'NONE', #1493, .T. ) ;
#9795=DIRECTION ( 'NONE',  ( 0.000000000000000000, 0.000000000000000000, 1.000000000000000000 ) ) ;
#9815=EDGE_LOOP ( 'NONE', ( #5633, #8652, #12284, #1386 ) ) ;
#9817=EDGE_CURVE ( 'NONE', #10905, #10264, #10717, .T. ) ;
#9825=CARTESIAN_POINT ( 'NONE',  ( 3.556430356250028790, 71.84604660189818048, 3.490625000614517415 ) ) ;
#9834=ORIENTED_EDGE ( 'NONE', *, *, #11090, .T. ) ;
#9836=CARTESIAN_POINT ( 'NONE',  ( 35.00000000000000000, 126.3079067962035822, 4.746875000614517504 ) ) ;
#9840=CARTESIAN_POINT ( 'NONE',  ( 3.800000000000015365, 90.00000000000000000, 3.762500001229034385 ) ) ;
#9843=DIRECTION ( 'NONE',  ( 0.000000000000000000, 0.000000000000000000, 1.000000000000000000 ) ) ;
#9847=CARTESIAN_POINT ( 'NONE',  ( 50.72178482187499071, 117.2309300971526937, 2.853125000614517237 ) ) ;
#9855=DIRECTION ( 'NONE',  ( 0.000000000000000000, 0.000000000000000000, -1.000000000000000000 ) ) ;
#9856=CARTESIAN_POINT ( 'NONE',  ( 3.556430356250015024, 90.00000000000000000, 4.859375000614517326 ) ) ;
#9862=LINE ( 'NONE', #890, #8572 ) ;
#9868=CARTESIAN_POINT ( 'NONE',  ( 3.800000000000055334, 71.98667160128364628, 4.137500000000000178 ) ) ;
#9869=CARTESIAN_POINT ( 'NONE',  ( 50.00000000000000000, 62.64236852357281293, -1.499999999999999778 ) ) ;
#9870=EDGE_CURVE ( 'NONE', #11286, #2819, #9192, .T. ) ;
#9880=VECTOR ( 'NONE', #6971, 1000.000000000000000 ) ;
#9882=DIRECTION ( 'NONE',  ( -0.000000000000000000, -0.000000000000000000, -1.000000000000000000 ) ) ;
#9884=CARTESIAN_POINT ( 'NONE',  ( 66.20000000000000284, 71.98667160128370313, 4.400000001229034119 ) ) ;
#9886=ADVANCED_FACE ( 'NONE', ( #2812 ), #12752, .T. ) ;
#9897=CARTESIAN_POINT ( 'NONE',  ( 3.556430356250014579, 108.1539533981018053, 4.371875000614517504 ) ) ;
#9900=CARTESIAN_POINT ( 'NONE',  ( 3.556430356250014579, 108.1539533981018053, 4.821875000614516793 ) ) ;
#9902=EDGE_CURVE ( 'NONE', #6195, #8482, #7311, .T. ) ;
#9941=CARTESIAN_POINT ( 'NONE',  ( 30.00000000000000711, 2.000000000000000000, -1.499999999999999556 ) ) ;
#9945=EDGE_LOOP ( 'NONE', ( #4015, #5765, #10671, #7941, #4109, #7651, #12570, #11122, #1256, #9619, #7256, #4372 ) ) ;
#9951=EDGE_CURVE ( 'NONE', #193, #10175, #9862, .T. ) ;
#9953=CARTESIAN_POINT ( 'NONE',  ( 66.19999999999998863, 90.00000000000000000, 3.987500001229034030 ) ) ;
#9956=ORIENTED_EDGE ( 'NONE', *, *, #12108, .F. ) ;
#9957=LINE ( 'NONE', #4861, #12648 ) ;
#9961=DIRECTION ( 'NONE',  ( -1.000000000000000000, 0.000000000000000000, 0.000000000000000000 ) ) ;
#9963=EDGE_CURVE ( 'NONE', #5827, #6538, #2684, .T. ) ;
#9965=CARTESIAN_POINT ( 'NONE',  ( 3.800000000000015365, 90.00000000000000000, 5.000000000000000000 ) ) ;
#9966=CARTESIAN_POINT ( 'NONE',  ( 3.556430356250028790, 71.84604660189818048, 3.040625000614517237 ) ) ;
#9967=ORIENTED_EDGE ( 'NONE', *, *, #2336, .T. ) ;
#9969=CARTESIAN_POINT ( 'NONE',  ( 66.20000000000004547, 108.0133283987162969, 3.575000001229034385 ) ) ;
#9976=CARTESIAN_POINT ( 'NONE',  ( 35.00000000000000000, 90.00000000000000000, 5.000000000000000000 ) ) ;
#9979=CARTESIAN_POINT ( 'NONE',  ( 40.00000000000000000, 0.000000000000000000, 10.00000000000000000 ) ) ;
#9986=AXIS2_PLACEMENT_3D ( 'NONE', #8028, #2805, #9855 ) ;
#9994=EDGE_CURVE ( 'NONE', #12910, #7130, #8185, .T. ) ;
#10001=DIRECTION ( 'NONE',  ( -0.000000000000000000, 1.000000000000000000, -0.000000000000000000 ) ) ;
#10009=ORIENTED_EDGE ( 'NONE', *, *, #4300, .F. ) ;
#10013=LINE ( 'NONE', #7792, #4838 ) ;
#10015=AXIS2_PLACEMENT_3D ( 'NONE', #7728, #4724, #6933 ) ;
#10016=CARTESIAN_POINT ( 'NONE',  ( 19.40000000000000924, 117.0199925980744666, 3.237500001229034030 ) ) ;
#10020=CARTESIAN_POINT ( 'NONE',  ( 60.43447242791587826, 111.3420572944792895, 3.026359441279048657 ) ) ;
#10025=VECTOR ( 'NONE', #1697, 1000.000000000000000 ) ;
#10029=CARTESIAN_POINT ( 'NONE',  ( 66.44356964374999563, 71.84604660189820891, 3.190625000614517592 ) ) ;
#10031=CARTESIAN_POINT ( 'NONE',  ( 50.72178482187499071, 117.2309300971526937, 4.709375000614516971 ) ) ;
#10053=ORIENTED_EDGE ( 'NONE', *, *, #12275, .F. ) ;
#10054=CARTESIAN_POINT ( 'NONE',  ( 30.00000000000000711, 90.00000000000000000, -8.000000000000000000 ) ) ;
#10060=DIRECTION ( 'NONE',  ( 0.000000000000000000, 0.000000000000000000, 1.000000000000000000 ) ) ;
#10062=ORIENTED_EDGE ( 'NONE', *, *, #2481, .T. ) ;
#10079=CARTESIAN_POINT ( 'NONE',  ( 50.72178482187501203, 62.76906990284730625, 4.559375000614517504 ) ) ;
#10082=ORIENTED_EDGE ( 'NONE', *, *, #516, .F. ) ;
#10085=ORIENTED_EDGE ( 'NONE', *, *, #7925, .T. ) ;
#10089=CARTESIAN_POINT ( 'NONE',  ( 19.27821517812503060, 62.76906990284727783, 3.528125000614517059 ) ) ;
#10097=CLOSED_SHELL ( 'NONE', ( #855, #8466, #759, #5906, #633, #7705, #3275, #556, #4449, #3767, #6899, #1342, #2396, #2489, #6138, #8721, #6943, #471, #5605, #3817, #8526, #7896, #9886, #8996, #7071, #1802, #9559, #7319, #9708, #11218, #12033, #9519, #6622, #2756, #4107, #4397, #4623, #3095, #11302, #548, #10201, #4610, #8418, #3682, #7650, #8233, #4034, #8222, #5362, #2731, #5070, #6415, #2531, #8601, #11433 ) ) ;
#10105=ORIENTED_EDGE ( 'NONE', *, *, #11744, .T. ) ;
#10108=AXIS2_PLACEMENT_3D ( 'NONE', #11143, #7291, #7160 ) ;
#10110=DIRECTION ( 'NONE',  ( -0.000000000000000000, 1.000000000000000000, 0.000000000000000000 ) ) ;
#10111=DIRECTION ( 'NONE',  ( -0.000000000000000000, 1.000000000000000000, -0.000000000000000000 ) ) ;
#10112=DIRECTION ( 'NONE',  ( 0.000000000000000000, 0.000000000000000000, 1.000000000000000000 ) ) ;
#10118=VERTEX_POINT ( 'NONE', #28 ) ;
#10119=ORIENTED_EDGE ( 'NONE', *, *, #9226, .F. ) ;
#10122=ORIENTED_EDGE ( 'NONE', *, *, #4912, .T. ) ;
#10138=EDGE_CURVE ( 'NONE', #3551, #7582, #5535, .T. ) ;
#10143=CARTESIAN_POINT ( 'NONE',  ( 3.800000000000025135, 71.98667160128366049, 2.900000001229034563 ) ) ;
#10144=SURFACE_STYLE_USAGE ( .BOTH. , #9779 ) ;
#10151=CARTESIAN_POINT ( 'NONE',  ( 66.19999999999997442, 108.0133283987163253, 3.912500000000000533 ) ) ;
#10159=CARTESIAN_POINT ( 'NONE',  ( 35.00000000000000711, 53.69209320379640360, 4.015625000614517326 ) ) ;
#10165=PRODUCT_DEFINITION ( 'UNKNOWN', '', #3849, #3210 ) ;
#10175=VERTEX_POINT ( 'NONE', #10314 ) ;
#10192=CARTESIAN_POINT ( 'NONE',  ( 66.19999999999998863, 90.00000000000000000, 4.437500001229033764 ) ) ;
#10199=CARTESIAN_POINT ( 'NONE',  ( 21.49999999999998579, 90.00000000000000000, -8.000000000000000000 ) ) ;
#10201=ADVANCED_FACE ( 'NONE', ( #6449 ), #1481, .T. ) ;
#10204=FACE_OUTER_BOUND ( 'NONE', #3719, .T. ) ;
#10206=EDGE_LOOP ( 'NONE', ( #8197, #7719, #6567, #12186 ) ) ;
#10214=EDGE_CURVE ( 'NONE', #6389, #8617, #5466, .T. ) ;
#10217=CARTESIAN_POINT ( 'NONE',  ( 35.00000000000000000, 126.0266567974326222, 3.987499999999999378 ) ) ;
#10225=CARTESIAN_POINT ( 'NONE',  ( 66.44356964374998142, 108.1539533981018053, 3.715625000614517948 ) ) ;
#10228=CARTESIAN_POINT ( 'NONE',  ( 19.27821517812500574, 117.2309300971526937, 3.434375000614517059 ) ) ;
#10244=ORIENTED_EDGE ( 'NONE', *, *, #11304, .F. ) ;
#10246=CARTESIAN_POINT ( 'NONE',  ( 3.800000000000015365, 90.00000000000000000, 4.549999999999999822 ) ) ;
#10257=CARTESIAN_POINT ( 'NONE',  ( 35.00000000000000000, 126.0266567974326222, 2.750000001229034208 ) ) ;
#10260=EDGE_CURVE ( 'NONE', #4053, #7731, #1494, .T. ) ;
#10264=VERTEX_POINT ( 'NONE', #11622 ) ;
#10268=CARTESIAN_POINT ( 'NONE',  ( 10.16381611175368604, 72.81849919625140899, -1.000000000000000000 ) ) ;
#10274=CARTESIAN_POINT ( 'NONE',  ( 50.59999999999999432, 117.0199925980744666, 2.712500001229034119 ) ) ;
#10278=CARTESIAN_POINT ( 'NONE',  ( 3.800000000000001155, 108.0133283987163111, 4.512500000000001066 ) ) ;
#10280=CARTESIAN_POINT ( 'NONE',  ( 3.556430356250015024, 90.00000000000000000, 4.409375000614517148 ) ) ;
#10284=CARTESIAN_POINT ( 'NONE',  ( 21.49999999999998579, 90.00000000000000000, -5.000000000000000000 ) ) ;
#10290=CARTESIAN_POINT ( 'NONE',  ( 3.556430356250014579, 108.1539533981018053, 3.471875000614516704 ) ) ;
#10304=ORIENTED_EDGE ( 'NONE', *, *, #9543, .F. ) ;
#10314=CARTESIAN_POINT ( 'NONE',  ( 66.19999999999998863, 90.00000000000000000, 3.425000000000000266 ) ) ;
#10318=CARTESIAN_POINT ( 'NONE',  ( 66.20000000000000284, 90.00000000000000000, -8.000000000000000000 ) ) ;
#10322=CARTESIAN_POINT ( 'NONE',  ( 50.59999999999999432, 117.0199925980744666, 2.712500001229034119 ) ) ;
#10324=CARTESIAN_POINT ( 'NONE',  ( 46.99999999999995737, 90.00000000000000000, -5.000000000000000000 ) ) ;
#10338=PLANE ( 'NONE',  #11464 ) ;
#10346=CARTESIAN_POINT ( 'NONE',  ( 19.27821517812503060, 62.76906990284727783, 3.134375000614517237 ) ) ;
#10351=VERTEX_POINT ( 'NONE', #3840 ) ;
#10358=CARTESIAN_POINT ( 'NONE',  ( 50.72178482187499071, 117.2309300971526937, 3.809375000614517504 ) ) ;
#10359=DIRECTION ( 'NONE',  ( -0.000000000000000000, -0.000000000000000000, -1.000000000000000000 ) ) ;
#10369=CARTESIAN_POINT ( 'NONE',  ( 50.59999999999999432, 117.0199925980744666, 4.850000000000000533 ) ) ;
#10378=EDGE_CURVE ( 'NONE', #3935, #12624, #1873, .T. ) ;
#10380=VERTEX_POINT ( 'NONE', #9658 ) ;
#10390=CARTESIAN_POINT ( 'NONE',  ( 35.00000000000000000, 126.0266567974326222, 4.550000001229034474 ) ) ;
#10401=ORIENTED_EDGE ( 'NONE', *, *, #10260, .T. ) ;
#10408=CARTESIAN_POINT ( 'NONE',  ( 66.20000000000008811, 108.0133283987162542, 3.125000001229034208 ) ) ;
#10421=CARTESIAN_POINT ( 'NONE',  ( 3.556430356250015024, 90.00000000000000000, 3.509375000614517681 ) ) ;
#10442=LINE ( 'NONE', #1411, #523 ) ;
#10443=FACE_BOUND ( 'NONE', #9212, .T. ) ;
#10451=ORIENTED_EDGE ( 'NONE', *, *, #1230, .F. ) ;
#10452=FACE_OUTER_BOUND ( 'NONE', #3493, .T. ) ;
#10467=VECTOR ( 'NONE', #12660, 1000.000000000000227 ) ;
#10473=VECTOR ( 'NONE', #8653, 1000.000000000000000 ) ;
#10474=CARTESIAN_POINT ( 'NONE',  ( 50.72178482187499071, 117.2309300971526937, 3.359375000614517326 ) ) ;
#10475=VERTEX_POINT ( 'NONE', #6966 ) ;
#10484=CARTESIAN_POINT ( 'NONE',  ( 3.556430356250015024, 90.00000000000000000, 4.409375000614517148 ) ) ;
#10486=CARTESIAN_POINT ( 'NONE',  ( 19.27821517812503060, 62.76906990284727783, 4.428125000614516971 ) ) ;
#10488=DIRECTION ( 'NONE',  ( -0.000000000000000000, -1.000000000000000000, -0.000000000000000000 ) ) ;
#10493=CARTESIAN_POINT ( 'NONE',  ( 25.00000000000000355, 2.000000000000001332, 4.150000000000012790 ) ) ;
#10517=AXIS2_PLACEMENT_3D ( 'NONE', #8198, #9170, #12185 ) ;
#10519=DIRECTION ( 'NONE',  ( -0.000000000000000000, -1.000000000000000000, -0.000000000000000000 ) ) ;
#10538=DIRECTION ( 'NONE',  ( 1.000000000000000000, 0.000000000000000000, -1.445602896647339656E-17 ) ) ;
#10543=CARTESIAN_POINT ( 'NONE',  ( 19.27821517812500574, 117.2309300971526937, 3.434375000614517059 ) ) ;
#10545=DIRECTION ( 'NONE',  ( 0.000000000000000000, 0.000000000000000000, 1.000000000000000000 ) ) ;
#10547=VERTEX_POINT ( 'NONE', #7098 ) ;
#10550=ORIENTED_EDGE ( 'NONE', *, *, #4912, .F. ) ;
#10561=DIRECTION ( 'NONE',  ( -0.000000000000000000, 1.000000000000000000, -0.000000000000000000 ) ) ;
#10579=ORIENTED_EDGE ( 'NONE', *, *, #301, .T. ) ;
#10593=( BOUNDED_SURFACE ( )  B_SPLINE_SURFACE ( 1, 2, ( 
 ( #9699, #3889, #7868, #11857, #4985, #735, #1052, #8260, #62, #7210, #5307, #127, #4334, #6225, #3098, #8131, #1253, #11258, #6154, #9035, #3296, #2047, #4142, #2179, #2313, #5246, #12117, #10217, #4207, #10151, #8323, #12250, #3164, #253, #4077, #5177, #7141, #11198, #3028, #8193, #1185, #10995, #9299, #7275, #7078, #9166, #2251, #1116, #6024, #5045, #190, #11123, #11059, #10020, #7015 ),
 ( #325, #5109, #12181, #8066, #12051, #2113, #9232, #6090, #10079, #3230, #4271, #6288, #10280, #1313, #9103, #7467, #12312, #2632, #6481, #9625, #4398, #6349, #5634, #11452, #8586, #2565, #2504, #5568, #7338, #4529, #11322, #11388, #1380, #586, #4658, #3360, #1511, #8453, #10543, #5497, #10474, #9495, #3420, #6544, #7402, #4592, #10346, #3552, #3618, #5368, #12577, #1578, #7596, #519, #651 ) ),
 .UNSPECIFIED., .F., .F., .F. ) 
 B_SPLINE_SURFACE_WITH_KNOTS ( ( 2, 2 ),
 ( 3, 2, 2, 2, 2, 2, 2, 2, 2, 2, 2, 2, 2, 2, 2, 2, 2, 2, 2, 2, 2, 2, 2, 2, 2, 2, 2, 3 ),
 ( 0.000000000000000000, 1.000000000000000000 ),
 ( 0.000000000000000000, 0.03333333333333333287, 0.06666666666666666574, 0.1000000000000000056, 0.1333333333333333315, 0.1666666666666666574, 0.2000000000000000111, 0.2333333333333333370, 0.2666666666666666630, 0.2999999999999999889, 0.3333333333333333148, 0.3666666666666666408, 0.4000000000000000222, 0.4333333333333333481, 0.4666666666666666741, 0.5000000000000000000, 0.5333333333333333259, 0.5666666666666666519, 0.5999999999999999778, 0.6333333333333333037, 0.6666666666666666297, 0.6999999999999999556, 0.7333333333333332815, 0.7666666666666667185, 0.8000000000000000444, 0.8333333333333333703, 0.8666666666666666963, 0.8887752010443024098 ),
 .UNSPECIFIED. ) 
 GEOMETRIC_REPRESENTATION_ITEM ( )  RATIONAL_B_SPLINE_SURFACE ( (
 ( 1.000000000000000000, 0.8660254037844387076, 1.000000000000000000, 0.8660254037844387076, 1.000000000000000000, 0.8660254037844387076, 1.000000000000000000, 0.8660254037844387076, 1.000000000000000000, 0.8660254037844387076, 1.000000000000000000, 0.8660254037844387076, 1.000000000000000000, 0.8660254037844387076, 1.000000000000000000, 0.8660254037844387076, 1.000000000000000000, 0.8660254037844387076, 1.000000000000000000, 0.8660254037844387076, 1.000000000000000000, 0.8660254037844387076, 1.000000000000000000, 0.8660254037844387076, 1.000000000000000000, 0.8660254037844387076, 1.000000000000000000, 0.8660254037844387076, 1.000000000000000000, 0.8660254037844387076, 1.000000000000000000, 0.8660254037844387076, 1.000000000000000000, 0.8660254037844387076, 1.000000000000000000, 0.8660254037844387076, 1.000000000000000000, 0.8660254037844387076, 1.000000000000000000, 0.8660254037844387076, 1.000000000000000000, 0.8660254037844387076, 1.000000000000000000, 0.8660254037844387076, 1.000000000000000000, 0.8660254037844387076, 1.000000000000000000, 0.8660254037844387076, 1.000000000000000000, 0.8660254037844387076, 1.000000000000000000, 0.8660254037844387076, 1.000000000000000000, 0.9111405410151519613, 0.9401542262549813511),
 ( 1.000000000000000000, 0.8660254037844387076, 1.000000000000000000, 0.8660254037844387076, 1.000000000000000000, 0.8660254037844387076, 1.000000000000000000, 0.8660254037844387076, 1.000000000000000000, 0.8660254037844387076, 1.000000000000000000, 0.8660254037844387076, 1.000000000000000000, 0.8660254037844387076, 1.000000000000000000, 0.8660254037844387076, 1.000000000000000000, 0.8660254037844387076, 1.000000000000000000, 0.8660254037844387076, 1.000000000000000000, 0.8660254037844387076, 1.000000000000000000, 0.8660254037844387076, 1.000000000000000000, 0.8660254037844387076, 1.000000000000000000, 0.8660254037844387076, 1.000000000000000000, 0.8660254037844387076, 1.000000000000000000, 0.8660254037844387076, 1.000000000000000000, 0.8660254037844387076, 1.000000000000000000, 0.8660254037844387076, 1.000000000000000000, 0.8660254037844387076, 1.000000000000000000, 0.8660254037844387076, 1.000000000000000000, 0.8660254037844387076, 1.000000000000000000, 0.8660254037844387076, 1.000000000000000000, 0.8660254037844387076, 1.000000000000000000, 0.8660254037844387076, 1.000000000000000000, 0.8660254037844387076, 1.000000000000000000, 0.8660254037844387076, 1.000000000000000000, 0.9111405410151519613, 0.9401542262549813511) ) ) 
 REPRESENTATION_ITEM ( '' )  SURFACE ( )  );
#10607=EDGE_CURVE ( 'NONE', #2423, #8376, #11345, .T. ) ;
#10608=ORIENTED_EDGE ( 'NONE', *, *, #1687, .F. ) ;
#10609=CARTESIAN_POINT ( 'NONE',  ( 3.800000000000039790, 71.98667160128364628, 4.250000001229034652 ) ) ;
#10615=CIRCLE ( 'NONE', #8932, 1.599999999999997202 ) ;
#10617=CARTESIAN_POINT ( 'NONE',  ( 20.00000000000000355, 2.000000000000000000, 1.499999999999999556 ) ) ;
#10622=CARTESIAN_POINT ( 'NONE',  ( 40.00000000000000000, 0.000000000000000000, 1.500000000000001332 ) ) ;
#10624=DIRECTION ( 'NONE',  ( -1.000000000000000000, 0.000000000000000000, 0.000000000000000000 ) ) ;
#10632=VERTEX_POINT ( 'NONE', #3445 ) ;
#10638=CARTESIAN_POINT ( 'NONE',  ( 66.44356964374999563, 90.00000000000000000, 3.228125000614517237 ) ) ;
#10642=ORIENTED_EDGE ( 'NONE', *, *, #5242, .F. ) ;
#10643=AXIS2_PLACEMENT_3D ( 'NONE', #5370, #2443, #1513 ) ;
#10658=ORIENTED_EDGE ( 'NONE', *, *, #8811, .F. ) ;
#10665=CIRCLE ( 'NONE', #11711, 31.19999999999998863 ) ;
#10667=ORIENTED_EDGE ( 'NONE', *, *, #7973, .T. ) ;
#10671=ORIENTED_EDGE ( 'NONE', *, *, #725, .F. ) ;
#10681=CARTESIAN_POINT ( 'NONE',  ( 35.00000000000000000, 126.0266567974326222, 4.100000001229034297 ) ) ;
#10689=CARTESIAN_POINT ( 'NONE',  ( 20.00000000000000355, 62.64236852357281293, -1.499999999999999556 ) ) ;
#10690=CARTESIAN_POINT ( 'NONE',  ( 66.44356964374999563, 71.84604660189820891, 3.246875000614517059 ) ) ;
#10696=CARTESIAN_POINT ( 'NONE',  ( 66.19999999999998863, 90.00000000000000000, 4.325000000000000178 ) ) ;
#10697=DIRECTION ( 'NONE',  ( -0.000000000000000000, -0.000000000000000000, -1.000000000000000000 ) ) ;
#10703=ORIENTED_EDGE ( 'NONE', *, *, #12475, .F. ) ;
#10706=VERTEX_POINT ( 'NONE', #4419 ) ;
#10711=CARTESIAN_POINT ( 'NONE',  ( 66.20000000000008811, 108.0133283987162542, 4.362499999999998934 ) ) ;
#10712=DIRECTION ( 'NONE',  ( -0.8660254037844400399, 0.000000000000000000, -0.4999999999999975575 ) ) ;
#10717=LINE ( 'NONE', #3859, #11276 ) ;
#10728=ORIENTED_EDGE ( 'NONE', *, *, #1911, .T. ) ;
#10735=DIRECTION ( 'NONE',  ( -1.000000000000000000, 0.000000000000000000, 0.000000000000000000 ) ) ;
#10738=VECTOR ( 'NONE', #6508, 1000.000000000000000 ) ;
#10740=CARTESIAN_POINT ( 'NONE',  ( 35.00000000000000000, 126.3079067962035822, 3.790625000614517237 ) ) ;
#10750=CARTESIAN_POINT ( 'NONE',  ( 64.54728993811707483, 100.7543353701752125, 2.858851390224067313 ) ) ;
#10752=CARTESIAN_POINT ( 'NONE',  ( 50.72178482187501203, 62.76906990284730625, 4.559375000614517504 ) ) ;
#10755=DIRECTION ( 'NONE',  ( 0.000000000000000000, 0.000000000000000000, 1.000000000000000000 ) ) ;
#10756=ORIENTED_EDGE ( 'NONE', *, *, #12549, .T. ) ;
#10759=( NAMED_UNIT ( * ) PLANE_ANGLE_UNIT ( ) SI_UNIT ( $, .RADIAN. ) );
#10764=VECTOR ( 'NONE', #12735, 1000.000000000000000 ) ;
#10766=CARTESIAN_POINT ( 'NONE',  ( 3.556430356250028790, 71.84604660189818048, 3.940625000614517592 ) ) ;
#10770=ORIENTED_EDGE ( 'NONE', *, *, #11229, .F. ) ;
#10771=FACE_OUTER_BOUND ( 'NONE', #11962, .T. ) ;
#10777=( BOUNDED_CURVE ( )  B_SPLINE_CURVE ( 2, ( #9342, #3399, #8235, #10257, #10322, #4314, #7377 ),
 .UNSPECIFIED., .F., .F. ) 
 B_SPLINE_CURVE_WITH_KNOTS ( ( 3, 2, 2, 3 ),
 ( 0.8000000000000002665, 0.8333333333333334814, 0.8666666666666666963, 0.8887752010635167066 ),
 .UNSPECIFIED. ) 
 CURVE ( )  GEOMETRIC_REPRESENTATION_ITEM ( )  RATIONAL_B_SPLINE_CURVE ( ( 0.9999999999999991118, 0.8660254037844395958, 1.000000000000000000, 0.8660254037844387076, 1.000000000000000000, 0.9111405409379251807, 0.9401542263054123438 ) ) 
 REPRESENTATION_ITEM ( '' )  );
#10779=CARTESIAN_POINT ( 'NONE',  ( 50.00000000000000000, 0.000000000000000000, 1.500000000000001332 ) ) ;
#10807=CARTESIAN_POINT ( 'NONE',  ( 35.00000000000000711, 53.97334320256736362, 3.875000001229034208 ) ) ;
#10818=VERTEX_POINT ( 'NONE', #3573 ) ;
#10820=CARTESIAN_POINT ( 'NONE',  ( 25.00000000000000355, 2.000000000000001332, 5.750000000000000000 ) ) ;
#10826=FACE_OUTER_BOUND ( 'NONE', #5876, .T. ) ;
#10827=CARTESIAN_POINT ( 'NONE',  ( 35.00000000000000000, 90.00000000000000000, -1.000000000000000000 ) ) ;
#10828=CARTESIAN_POINT ( 'NONE',  ( 66.44356964375000985, 71.84604660189820891, 4.090625000614517504 ) ) ;
#10832=VERTEX_POINT ( 'NONE', #10689 ) ;
#10833=EDGE_CURVE ( 'NONE', #9108, #1636, #7684, .T. ) ;
#10838=LINE ( 'NONE', #12935, #8429 ) ;
#10848=EDGE_CURVE ( 'NONE', #2423, #10475, #11512, .T. ) ;
#10849=VECTOR ( 'NONE', #9163, 1000.000000000000000 ) ;
#10851=ORIENTED_EDGE ( 'NONE', *, *, #516, .T. ) ;
#10853=LINE ( 'NONE', #6732, #2280 ) ;
#10864=CARTESIAN_POINT ( 'NONE',  ( 25.00000000000000355, 2.000000000000001332, -5.750000000000000000 ) ) ;
#10866=CARTESIAN_POINT ( 'NONE',  ( 3.556430356250028790, 71.84604660189818048, 3.040625000614517237 ) ) ;
#10879=CARTESIAN_POINT ( 'NONE',  ( 3.556430356250014579, 108.1539533981018053, 3.471875000614516704 ) ) ;
#10893=DIRECTION ( 'NONE',  ( -1.000000000000000000, 0.000000000000000000, -0.000000000000000000 ) ) ;
#10896=CARTESIAN_POINT ( 'NONE',  ( 3.800000000000015365, 90.00000000000000000, 4.662500001229034297 ) ) ;
#10898=EDGE_CURVE ( 'NONE', #4053, #7376, #2656, .T. ) ;
#10905=VERTEX_POINT ( 'NONE', #6693 ) ;
#10909=ORIENTED_EDGE ( 'NONE', *, *, #2035, .F. ) ;
#10912=ORIENTED_EDGE ( 'NONE', *, *, #6683, .T. ) ;
#10913=CIRCLE ( 'NONE', #9246, 1.599999999999990319 ) ;
#10921=EDGE_LOOP ( 'NONE', ( #7407, #11863 ) ) ;
#10923=CARTESIAN_POINT ( 'NONE',  ( 48.49999999999995737, 90.00000000000000000, -8.000000000000000000 ) ) ;
#10926=CARTESIAN_POINT ( 'NONE',  ( 3.556430356250015024, 90.00000000000000000, 3.453125000614517770 ) ) ;
#10927=AXIS2_PLACEMENT_3D ( 'NONE', #6214, #7065, #179 ) ;
#10938=LINE ( 'NONE', #9965, #5862 ) ;
#10939=CARTESIAN_POINT ( 'NONE',  ( 35.00000000000000000, 126.3079067962035822, 4.296875000614517326 ) ) ;
#10940=ORIENTED_EDGE ( 'NONE', *, *, #5856, .F. ) ;
#10944=DIRECTION ( 'NONE',  ( -0.000000000000000000, 1.000000000000000000, -0.000000000000000000 ) ) ;
#10949=DIRECTION ( 'NONE',  ( 0.000000000000000000, 0.000000000000000000, 1.000000000000000000 ) ) ;
#10950=CARTESIAN_POINT ( 'NONE',  ( 35.00000000000000000, 90.00000000000000000, -5.000000000000000000 ) ) ;
#10955=CIRCLE ( 'NONE', #9713, 1.599999999999986766 ) ;
#10961=DIRECTION ( 'NONE',  ( 1.000000000000000000, 0.000000000000000000, 0.000000000000000000 ) ) ;
#10964=AXIS2_PLACEMENT_3D ( 'NONE', #1496, #3346, #2424 ) ;
#10967=CARTESIAN_POINT ( 'NONE',  ( 35.00000000000000000, 126.0266567974326222, 4.100000001229034297 ) ) ;
#10973=( GEOMETRIC_REPRESENTATION_CONTEXT ( 3 ) GLOBAL_UNCERTAINTY_ASSIGNED_CONTEXT ( ( #1082 ) ) GLOBAL_UNIT_ASSIGNED_CONTEXT ( ( #4451, #6470, #3733 ) ) REPRESENTATION_CONTEXT ( 'NONE', 'WORKASPACE' ) );
#10991=FILL_AREA_STYLE_COLOUR ( '', #9266 ) ;
#10995=CARTESIAN_POINT ( 'NONE',  ( 66.19999999999997442, 108.0133283987163253, 3.462499999999999911 ) ) ;
#11002=DIRECTION ( 'NONE',  ( 0.000000000000000000, 0.000000000000000000, -1.000000000000000000 ) ) ;
#11003=CARTESIAN_POINT ( 'NONE',  ( 35.00000000000000000, 126.3079067962035822, 4.240625000614517859 ) ) ;
#11018=ORIENTED_EDGE ( 'NONE', *, *, #5108, .F. ) ;
#11022=CARTESIAN_POINT ( 'NONE',  ( 3.800000000000015365, 90.00000000000000000, 4.212500001229034119 ) ) ;
#11046=AXIS2_PLACEMENT_3D ( 'NONE', #1113, #5105, #9100 ) ;
#11054=AXIS2_PLACEMENT_3D ( 'NONE', #12376, #5435, #10545 ) ;
#11059=CARTESIAN_POINT ( 'NONE',  ( 50.59999999999999432, 117.0199925980744666, 3.050000000000000266 ) ) ;
#11066=DIRECTION ( 'NONE',  ( -0.000000000000000000, -1.000000000000000000, -0.000000000000000000 ) ) ;
#11067=EDGE_CURVE ( 'NONE', #12910, #108, #10938, .T. ) ;
#11070=CARTESIAN_POINT ( 'NONE',  ( 3.556430356250014579, 108.1539533981018053, 3.865625000614517415 ) ) ;
#11078=EDGE_CURVE ( 'NONE', #2817, #4053, #1, .T. ) ;
#11081=VECTOR ( 'NONE', #11002, 1000.000000000000000 ) ;
#11090=EDGE_CURVE ( 'NONE', #5692, #10905, #2257, .T. ) ;
#11109=ORIENTED_EDGE ( 'NONE', *, *, #7973, .F. ) ;
#11122=ORIENTED_EDGE ( 'NONE', *, *, #2370, .F. ) ;
#11123=CARTESIAN_POINT ( 'NONE',  ( 35.00000000000000000, 126.0266567974326222, 3.087499999999999911 ) ) ;
#11125=DIRECTION ( 'NONE',  ( 0.000000000000000000, 0.000000000000000000, 1.000000000000000000 ) ) ;
#11130=FACE_OUTER_BOUND ( 'NONE', #3873, .T. ) ;
#11133=CARTESIAN_POINT ( 'NONE',  ( 3.556430356250014579, 108.1539533981018053, 3.415625000614517237 ) ) ;
#11134=ORIENTED_EDGE ( 'NONE', *, *, #11744, .F. ) ;
#11136=CARTESIAN_POINT ( 'NONE',  ( 5.011331584521383498, 81.39071625125095011, 5.000000000000000000 ) ) ;
#11143=CARTESIAN_POINT ( 'NONE',  ( 48.49999999999995737, 90.00000000000000000, -5.000000000000000000 ) ) ;
#11147=PLANE ( 'NONE',  #123 ) ;
#11148=ORIENTED_EDGE ( 'NONE', *, *, #11340, .F. ) ;
#11162=DIRECTION ( 'NONE',  ( -1.000000000000000000, 0.000000000000000000, 0.000000000000000000 ) ) ;
#11165=ORIENTED_EDGE ( 'NONE', *, *, #12642, .T. ) ;
#11177=CYLINDRICAL_SURFACE ( 'NONE', #1362, 30.19999999999998863 ) ;
#11181=EDGE_CURVE ( 'NONE', #6728, #5916, #8384, .T. ) ;
#11186=CARTESIAN_POINT ( 'NONE',  ( 0.000000000000000000, 0.000000000000000000, 10.00000000000000000 ) ) ;
#11192=CARTESIAN_POINT ( 'NONE',  ( 35.00000000000000711, 53.97334320256736362, 2.975000001229034741 ) ) ;
#11198=CARTESIAN_POINT ( 'NONE',  ( 3.800000000000015365, 108.0133283987163111, 3.612500000000000711 ) ) ;
#11204=ORIENTED_EDGE ( 'NONE', *, *, #1425, .T. ) ;
#11206=CARTESIAN_POINT ( 'NONE',  ( 66.44356964374999563, 90.00000000000000000, 3.228125000614517237 ) ) ;
#11208=CARTESIAN_POINT ( 'NONE',  ( 3.556430356250028790, 71.84604660189818048, 3.996875000614517504 ) ) ;
#11211=DIRECTION ( 'NONE',  ( 0.000000000000000000, 0.000000000000000000, 1.000000000000000000 ) ) ;
#11218=ADVANCED_FACE ( 'NONE', ( #11130 ), #9433, .T. ) ;
#11222=VECTOR ( 'NONE', #9388, 1000.000000000000000 ) ;
#11229=EDGE_CURVE ( 'NONE', #8114, #6389, #1690, .T. ) ;
#11249=LINE ( 'NONE', #5359, #6037 ) ;
#11254=CARTESIAN_POINT ( 'NONE',  ( 50.59999999999999432, 117.0199925980744666, 3.162500001229034741 ) ) ;
#11258=CARTESIAN_POINT ( 'NONE',  ( 66.19999999999997442, 108.0133283987163253, 4.362499999999999822 ) ) ;
#11270=CARTESIAN_POINT ( 'NONE',  ( 40.00000000000000000, 0.000000000000000000, 10.00000000000000000 ) ) ;
#11271=LINE ( 'NONE', #2325, #6428 ) ;
#11276=VECTOR ( 'NONE', #1757, 1000.000000000000000 ) ;
#11279=CARTESIAN_POINT ( 'NONE',  ( 30.00000000000000711, 0.000000000000000000, 10.00000000000000000 ) ) ;
#11286=VERTEX_POINT ( 'NONE', #2770 ) ;
#11298=ORIENTED_EDGE ( 'NONE', *, *, #7437, .F. ) ;
#11300=VECTOR ( 'NONE', #6474, 1000.000000000000000 ) ;
#11302=ADVANCED_FACE ( 'NONE', ( #9568 ), #9633, .F. ) ;
#11303=ORIENTED_EDGE ( 'NONE', *, *, #6631, .F. ) ;
#11304=EDGE_CURVE ( 'NONE', #3688, #11641, #6681, .T. ) ;
#11314=CARTESIAN_POINT ( 'NONE',  ( 30.00000000000000711, 2.000000000000000000, -10.00000000000000000 ) ) ;
#11318=EDGE_CURVE ( 'NONE', #108, #4396, #2841, .T. ) ;
#11322=CARTESIAN_POINT ( 'NONE',  ( 66.44356964374999563, 90.00000000000000000, 3.734375000614516882 ) ) ;
#11323=ORIENTED_EDGE ( 'NONE', *, *, #12302, .F. ) ;
#11331=CARTESIAN_POINT ( 'NONE',  ( 66.44356964374998142, 108.1539533981018053, 3.771875000614516082 ) ) ;
#11332=CARTESIAN_POINT ( 'NONE',  ( 66.44356964374999563, 90.00000000000000000, 4.578125000614516438 ) ) ;
#11340=EDGE_CURVE ( 'NONE', #10832, #2101, #5506, .T. ) ;
#11345=( BOUNDED_CURVE ( )  B_SPLINE_CURVE ( 2, ( #2270, #9448, #12392, #473, #10369, #2524, #3509 ),
 .UNSPECIFIED., .F., .F. ) 
 B_SPLINE_CURVE_WITH_KNOTS ( ( 3, 2, 2, 3 ),
 ( 0.000000000000000000, 0.03333333333333339532, 0.06666666666666679064, 0.1000000000000001860 ),
 .UNSPECIFIED. ) 
 CURVE ( )  GEOMETRIC_REPRESENTATION_ITEM ( )  RATIONAL_B_SPLINE_CURVE ( ( 1.000000000000000000, 0.8660254037844387076, 1.000000000000000000, 0.8660254037844387076, 1.000000000000000000, 0.8660254037844380415, 1.000000000000000666 ) ) 
 REPRESENTATION_ITEM ( '' )  );
#11351=LINE ( 'NONE', #5395, #3440 ) ;
#11354=( GEOMETRIC_REPRESENTATION_CONTEXT ( 3 ) GLOBAL_UNCERTAINTY_ASSIGNED_CONTEXT ( ( #4655 ) ) GLOBAL_UNIT_ASSIGNED_CONTEXT ( ( #3024, #10759, #3160 ) ) REPRESENTATION_CONTEXT ( 'NONE', 'WORKASPACE' ) );
#11355=ORIENTED_EDGE ( 'NONE', *, *, #4413, .F. ) ;
#11364=ORIENTED_EDGE ( 'NONE', *, *, #739, .T. ) ;
#11370=CARTESIAN_POINT ( 'NONE',  ( 4.800000000000015810, 90.00000000000000000, -5.000000000000000000 ) ) ;
#11384=CARTESIAN_POINT ( 'NONE',  ( 66.19999999999988916, 71.98667160128361786, 4.737499999999998934 ) ) ;
#11385=DIRECTION ( 'NONE',  ( 1.445602896647339656E-17, -0.000000000000000000, 1.000000000000000000 ) ) ;
#11388=CARTESIAN_POINT ( 'NONE',  ( 66.44356964374999563, 71.84604660189820891, 3.696875000614517237 ) ) ;
#11391=FACE_BOUND ( 'NONE', #2895, .T. ) ;
#11392=AXIS2_PLACEMENT_3D ( 'NONE', #1036, #6008, #4190 ) ;
#11399=CARTESIAN_POINT ( 'NONE',  ( 50.72178482187499071, 117.2309300971526937, 3.359375000614517326 ) ) ;
#11408=EDGE_CURVE ( 'NONE', #5251, #8056, #1517, .T. ) ;
#11418=DIRECTION ( 'NONE',  ( -0.000000000000000000, -0.000000000000000000, 1.000000000000000000 ) ) ;
#11421=CARTESIAN_POINT ( 'NONE',  ( 21.49999999999998579, 90.00000000000000000, -8.000000000000000000 ) ) ;
#11422=CARTESIAN_POINT ( 'NONE',  ( 4.800000000000015810, 90.00000000000000000, 5.000000000000000000 ) ) ;
#11428=FACE_BOUND ( 'NONE', #10921, .T. ) ;
#11433=ADVANCED_FACE ( 'NONE', ( #6938 ), #7069, .F. ) ;
#11448=CARTESIAN_POINT ( 'NONE',  ( 66.19999999999998863, 90.00000000000000000, 4.774999999999999467 ) ) ;
#11449=CARTESIAN_POINT ( 'NONE',  ( 45.00000000000000000, 0.000000000000000000, 5.750000000000000888 ) ) ;
#11451=VERTEX_POINT ( 'NONE', #2038 ) ;
#11452=CARTESIAN_POINT ( 'NONE',  ( 3.556430356250028790, 71.84604660189818048, 3.996875000614517059 ) ) ;
#11455=CARTESIAN_POINT ( 'NONE',  ( 3.799999999999904787, 71.98667160128373155, 2.900000001229034563 ) ) ;
#11457=ORIENTED_EDGE ( 'NONE', *, *, #11951, .T. ) ;
#11461=DIRECTION ( 'NONE',  ( 0.000000000000000000, 0.000000000000000000, 1.000000000000000000 ) ) ;
#11462=CARTESIAN_POINT ( 'NONE',  ( 35.00000000000000711, 53.69209320379639649, 3.171875000614517326 ) ) ;
#11464=AXIS2_PLACEMENT_3D ( 'NONE', #11186, #6215, #245 ) ;
#11465=DIRECTION ( 'NONE',  ( -0.000000000000000000, 1.000000000000000000, -0.000000000000000000 ) ) ;
#11472=VECTOR ( 'NONE', #4158, 1000.000000000000000 ) ;
#11484=DIRECTION ( 'NONE',  ( 0.000000000000000000, 0.000000000000000000, -1.000000000000000000 ) ) ;
#11487=EDGE_LOOP ( 'NONE', ( #10642, #2208, #1033, #5488 ) ) ;
#11488=DIRECTION ( 'NONE',  ( -1.000000000000000000, 0.000000000000000000, 0.000000000000000000 ) ) ;
#11493=FACE_OUTER_BOUND ( 'NONE', #8852, .T. ) ;
#11496=DIRECTION ( 'NONE',  ( -0.000000000000000000, -0.000000000000000000, -1.000000000000000000 ) ) ;
#11500=ORIENTED_EDGE ( 'NONE', *, *, #7265, .T. ) ;
#11511=EDGE_CURVE ( 'NONE', #4218, #3842, #10013, .T. ) ;
#11512=CIRCLE ( 'NONE', #6280, 31.19999999999999218 ) ;
#11517=EDGE_CURVE ( 'NONE', #4278, #9690, #12776, .T. ) ;
#11520=CARTESIAN_POINT ( 'NONE',  ( 50.60000000000001563, 62.98000740192552627, 4.362500001229034474 ) ) ;
#11522=APPLICATION_CONTEXT ( 'automotive_design' ) ;
#11535=CARTESIAN_POINT ( 'NONE',  ( 3.800000000000015365, 90.00000000000000000, 4.831250000614517148 ) ) ;
#11549=CARTESIAN_POINT ( 'NONE',  ( 22.99999999999998579, 90.00000000000000000, -8.000000000000000000 ) ) ;
#11550=PLANE ( 'NONE',  #1373 ) ;
#11560=DIRECTION ( 'NONE',  ( 0.000000000000000000, -1.000000000000000000, 0.000000000000000000 ) ) ;
#11569=CYLINDRICAL_SURFACE ( 'NONE', #10964, 1.500000000000001332 ) ;
#11577=ORIENTED_EDGE ( 'NONE', *, *, #4317, .T. ) ;
#11605=CARTESIAN_POINT ( 'NONE',  ( 45.00000000000000000, 0.000000000000000000, 7.349999999999997868 ) ) ;
#11609=AXIS2_PLACEMENT_3D ( 'NONE', #10827, #4942, #11746 ) ;
#11620=DIRECTION ( 'NONE',  ( 0.8660254037844365982, 0.5000000000000036637, 0.000000000000000000 ) ) ;
#11622=CARTESIAN_POINT ( 'NONE',  ( 50.00000000000000000, 2.000000000000000000, -10.00000000000000000 ) ) ;
#11628=VECTOR ( 'NONE', #7425, 1000.000000000000000 ) ;
#11635=DIRECTION ( 'NONE',  ( -0.000000000000000000, 1.000000000000000000, -0.000000000000000000 ) ) ;
#11637=CARTESIAN_POINT ( 'NONE',  ( 30.00000000000000711, 0.000000000000000000, 10.00000000000000000 ) ) ;
#11640=AXIS2_PLACEMENT_3D ( 'NONE', #9979, #3057, #8807 ) ;
#11641=VERTEX_POINT ( 'NONE', #11314 ) ;
#11657=CARTESIAN_POINT ( 'NONE',  ( 35.00000000000000000, 126.0266567974326222, 3.987500000000000266 ) ) ;
#11658=CARTESIAN_POINT ( 'NONE',  ( 20.00000000000000355, 0.000000000000000000, 1.500000000000000444 ) ) ;
#11660=CARTESIAN_POINT ( 'NONE',  ( 60.63303222545420823, 111.5086687406912347, 2.829484441871016109 ) ) ;
#11665=CARTESIAN_POINT ( 'NONE',  ( 3.800000000000015365, 90.00000000000000000, 3.762500001229034385 ) ) ;
#11668=DIRECTION ( 'NONE',  ( -1.000000000000000000, 0.000000000000000000, 0.000000000000000000 ) ) ;
#11670=CARTESIAN_POINT ( 'NONE',  ( 35.00000000000000000, 126.3079067962035822, 3.396875000614517415 ) ) ;
#11683=CARTESIAN_POINT ( 'NONE',  ( 3.556430356250014579, 108.1539533981018053, 3.865625000614517415 ) ) ;
#11692=SHAPE_REPRESENTATION ( 'wheel support and navigator', ( #5704 ), #11354 ) ;
#11698=ORIENTED_EDGE ( 'NONE', *, *, #1510, .T. ) ;
#11703=DIRECTION ( 'NONE',  ( -0.000000000000000000, -0.000000000000000000, 1.000000000000000000 ) ) ;
#11706=CARTESIAN_POINT ( 'NONE',  ( 64.31840935109022439, 100.6710296186405742, 2.661976390793298286 ) ) ;
#11711=AXIS2_PLACEMENT_3D ( 'NONE', #8755, #1820, #9669 ) ;
#11715=FACE_BOUND ( 'NONE', #1684, .T. ) ;
#11724=CARTESIAN_POINT ( 'NONE',  ( 3.800000000000025135, 71.98667160128366049, 4.250000001229034652 ) ) ;
#11730=DIRECTION ( 'NONE',  ( 1.000000000000000000, -0.000000000000000000, -0.000000000000000000 ) ) ;
#11733=CARTESIAN_POINT ( 'NONE',  ( 66.44356964374999563, 90.00000000000000000, 3.284375000614517148 ) ) ;
#11744=EDGE_CURVE ( 'NONE', #6635, #716, #709, .T. ) ;
#11746=DIRECTION ( 'NONE',  ( 1.000000000000000000, 0.000000000000000000, 0.000000000000000000 ) ) ;
#11747=CARTESIAN_POINT ( 'NONE',  ( 3.556430356250028790, 71.84604660189818048, 3.040625000614517681 ) ) ;
#11752=FACE_BOUND ( 'NONE', #6286, .T. ) ;
#11757=LINE ( 'NONE', #1818, #5292 ) ;
#11766=CIRCLE ( 'NONE', #7385, 1.500000000000001332 ) ;
#11768=ORIENTED_EDGE ( 'NONE', *, *, #1687, .T. ) ;
#11772=( GEOMETRIC_REPRESENTATION_CONTEXT ( 3 ) GLOBAL_UNCERTAINTY_ASSIGNED_CONTEXT ( ( #7659 ) ) GLOBAL_UNIT_ASSIGNED_CONTEXT ( ( #2044, #5173, #9161 ) ) REPRESENTATION_CONTEXT ( 'NONE', 'WORKASPACE' ) );
#11774=VECTOR ( 'NONE', #3981, 1000.000000000000000 ) ;
#11781=VERTEX_POINT ( 'NONE', #11706 ) ;
#11790=CARTESIAN_POINT ( 'NONE',  ( 19.40000000000000924, 117.0199925980744666, 4.587500001229034119 ) ) ;
#11792=DIRECTION ( 'NONE',  ( -0.000000000000000000, -0.000000000000000000, -1.000000000000000000 ) ) ;
#11793=DIRECTION ( 'NONE',  ( -0.000000000000000000, -0.000000000000000000, -1.000000000000000000 ) ) ;
#11804=CARTESIAN_POINT ( 'NONE',  ( 19.27821517812500574, 117.2309300971526937, 3.434375000614517059 ) ) ;
#11812=FACE_BOUND ( 'NONE', #12415, .T. ) ;
#11815=CARTESIAN_POINT ( 'NONE',  ( 35.00000000000000711, 53.69209320379639649, 3.115625000614517415 ) ) ;
#11821=ORIENTED_EDGE ( 'NONE', *, *, #12762, .T. ) ;
#11832=ORIENTED_EDGE ( 'NONE', *, *, #1331, .T. ) ;
#11838=EDGE_CURVE ( 'NONE', #6325, #10905, #12025, .T. ) ;
#11841=ORIENTED_EDGE ( 'NONE', *, *, #9951, .F. ) ;
#11845=FACE_BOUND ( 'NONE', #6583, .T. ) ;
#11848=VERTEX_POINT ( 'NONE', #9010 ) ;
#11852=CARTESIAN_POINT ( 'NONE',  ( 19.40000000000002700, 62.98000740192551206, 3.387500001229033941 ) ) ;
#11853=CARTESIAN_POINT ( 'NONE',  ( 3.556430356250015024, 90.00000000000000000, 3.003125000614517148 ) ) ;
#11857=CARTESIAN_POINT ( 'NONE',  ( 35.00000000000000000, 126.0266567974326222, 4.887500000000001066 ) ) ;
#11860=VECTOR ( 'NONE', #9311, 1000.000000000000000 ) ;
#11863=ORIENTED_EDGE ( 'NONE', *, *, #12466, .F. ) ;
#11865=CARTESIAN_POINT ( 'NONE',  ( 66.44356964374999563, 71.84604660189820891, 4.596875000614517148 ) ) ;
#11876=DIRECTION ( 'NONE',  ( 0.000000000000000000, 0.000000000000000000, 1.000000000000000000 ) ) ;
#11881=CARTESIAN_POINT ( 'NONE',  ( 35.00000000000000000, 90.00000000000000000, -5.000000000000000000 ) ) ;
#11891=CARTESIAN_POINT ( 'NONE',  ( 35.00000000000000000, 90.00000000000000000, -8.000000000000000000 ) ) ;
#11899=LINE ( 'NONE', #7055, #3405 ) ;
#11902=EDGE_LOOP ( 'NONE', ( #5824, #4929 ) ) ;
#11916=CARTESIAN_POINT ( 'NONE',  ( 19.40000000000000924, 117.0199925980744666, 4.137500001229033941 ) ) ;
#11925=( BOUNDED_CURVE ( )  B_SPLINE_CURVE ( 2, ( #1645, #8391, #11520, #6610, #12442, #10609, #6413 ),
 .UNSPECIFIED., .F., .F. ) 
 B_SPLINE_CURVE_WITH_KNOTS ( ( 3, 2, 2, 3 ),
 ( 0.1000000000000001860, 0.1333333333333334425, 0.1666666666666666852, 0.2000000000000000111 ),
 .UNSPECIFIED. ) 
 CURVE ( )  GEOMETRIC_REPRESENTATION_ITEM ( )  RATIONAL_B_SPLINE_CURVE ( ( 0.9999999999999992228, 0.8660254037844394848, 1.000000000000000000, 0.8660254037844387076, 1.000000000000000000, 0.8660254037844388186, 0.9999999999999998890 ) ) 
 REPRESENTATION_ITEM ( '' )  );
#11929=CARTESIAN_POINT ( 'NONE',  ( 50.72178482187499071, 117.2309300971526937, 4.709375000614516971 ) ) ;
#11930=EDGE_CURVE ( 'NONE', #6209, #5251, #4485, .T. ) ;
#11945=PLANE ( 'NONE',  #9986 ) ;
#11951=EDGE_CURVE ( 'NONE', #1608, #5251, #5219, .T. ) ;
#11953=AXIS2_PLACEMENT_3D ( 'NONE', #1977, #4009, #11976 ) ;
#11962=EDGE_LOOP ( 'NONE', ( #3829, #1509 ) ) ;
#11964=ORIENTED_EDGE ( 'NONE', *, *, #3108, .T. ) ;
#11965=B_SPLINE_CURVE_WITH_KNOTS ( 'NONE', 3,
 ( #3825, #3034, #4738, #10750 ),
 .UNSPECIFIED., .F., .F.,
 ( 4, 4 ),
 ( 0.000000000000000000, 1.000000000000000000 ),
 .UNSPECIFIED. ) ;
#11971=CARTESIAN_POINT ( 'NONE',  ( 20.00000000000000355, 2.000000000000000000, 10.00000000000000000 ) ) ;
#11974=DIRECTION ( 'NONE',  ( 0.000000000000000000, 0.000000000000000000, 1.000000000000000000 ) ) ;
#11976=DIRECTION ( 'NONE',  ( -1.000000000000000000, 0.000000000000000000, 0.000000000000000000 ) ) ;
#11977=CARTESIAN_POINT ( 'NONE',  ( 35.00000000000000000, 126.0266567974326222, 3.650000001229034119 ) ) ;
#11980=CARTESIAN_POINT ( 'NONE',  ( 64.54728993811707483, 100.7543353701752125, 2.858851390224067313 ) ) ;
#11987=CARTESIAN_POINT ( 'NONE',  ( 3.800000000000015365, 90.00000000000000000, 5.000000000000000000 ) ) ;
#11989=CARTESIAN_POINT ( 'NONE',  ( 3.556430356250015024, 90.00000000000000000, 4.831250000614517148 ) ) ;
#11990=CARTESIAN_POINT ( 'NONE',  ( 50.72178482187499071, 117.2309300971526937, 3.753125000614517592 ) ) ;
#11991=ORIENTED_EDGE ( 'NONE', *, *, #6960, .T. ) ;
#11994=LINE ( 'NONE', #8983, #5996 ) ;
#12000=CARTESIAN_POINT ( 'NONE',  ( 64.54728994471078352, 100.7543353520590870, 2.802601390178781404 ) ) ;
#12007=ORIENTED_EDGE ( 'NONE', *, *, #9072, .T. ) ;
#12014=CIRCLE ( 'NONE', #1571, 1.500000000000001332 ) ;
#12023=CARTESIAN_POINT ( 'NONE',  ( 50.00000000000000000, 2.000000000000000000, -10.00000000000000000 ) ) ;
#12025=LINE ( 'NONE', #3864, #862 ) ;
#12028=CARTESIAN_POINT ( 'NONE',  ( 35.00000000000000711, 53.97334320256736362, 4.212500000000000355 ) ) ;
#12032=EDGE_CURVE ( 'NONE', #2817, #6997, #7266, .T. ) ;
#12033=ADVANCED_FACE ( 'NONE', ( #9505 ), #4219, .F. ) ;
#12051=CARTESIAN_POINT ( 'NONE',  ( 50.72178482187499071, 117.2309300971526937, 4.709375000614516971 ) ) ;
#12055=CARTESIAN_POINT ( 'NONE',  ( 66.19999999999993179, 71.98667160128364628, 3.837499999999999911 ) ) ;
#12057=AXIS2_PLACEMENT_3D ( 'NONE', #6810, #4855, #1782 ) ;
#12060=CARTESIAN_POINT ( 'NONE',  ( 3.556430356250015024, 90.00000000000000000, 3.003125000614517148 ) ) ;
#12076=ORIENTED_EDGE ( 'NONE', *, *, #12308, .T. ) ;
#12081=VECTOR ( 'NONE', #10519, 1000.000000000000000 ) ;
#12108=EDGE_CURVE ( 'NONE', #2190, #10351, #4235, .T. ) ;
#12111=CARTESIAN_POINT ( 'NONE',  ( 3.800000000000015365, 90.00000000000000000, 3.312500001229034652 ) ) ;
#12117=CARTESIAN_POINT ( 'NONE',  ( 19.40000000000000924, 117.0199925980744666, 4.025000000000000355 ) ) ;
#12120=VERTEX_POINT ( 'NONE', #3752 ) ;
#12122=FACE_OUTER_BOUND ( 'NONE', #4721, .T. ) ;
#12132=CARTESIAN_POINT ( 'NONE',  ( 45.00000000000000000, 2.000000000000001332, -4.150000000000009237 ) ) ;
#12148=CARTESIAN_POINT ( 'NONE',  ( 35.00000000000000000, 90.00000000000000000, 1.000000000000000000 ) ) ;
#12151=CARTESIAN_POINT ( 'NONE',  ( 19.40000000000000924, 117.0199925980744666, 4.137500001229033941 ) ) ;
#12176=AXIS2_PLACEMENT_3D ( 'NONE', #9681, #2693, #776 ) ;
#12181=CARTESIAN_POINT ( 'NONE',  ( 19.27821517812500574, 117.2309300971526937, 4.784375000614516260 ) ) ;
#12185=DIRECTION ( 'NONE',  ( -1.000000000000000000, 0.000000000000000000, 0.000000000000000000 ) ) ;
#12186=ORIENTED_EDGE ( 'NONE', *, *, #6067, .F. ) ;
#12189=CARTESIAN_POINT ( 'NONE',  ( 19.27821517812503060, 62.76906990284727783, 3.978125000614516793 ) ) ;
#12191=DIRECTION ( 'NONE',  ( 1.000000000000000000, 0.000000000000000000, 0.000000000000000000 ) ) ;
#12193=DIRECTION ( 'NONE',  ( 0.000000000000000000, 0.000000000000000000, 1.000000000000000000 ) ) ;
#12226=CARTESIAN_POINT ( 'NONE',  ( 64.47099661891824951, 100.7265662098817955, 2.755726390383620217 ) ) ;
#12237=CIRCLE ( 'NONE', #11609, 30.19999999999999218 ) ;
#12238=CARTESIAN_POINT ( 'NONE',  ( 30.00000000000000711, 2.000000000000001776, 1.500000000000000666 ) ) ;
#12240=EDGE_LOOP ( 'NONE', ( #9353, #8170, #9593, #8140 ) ) ;
#12245=CARTESIAN_POINT ( 'NONE',  ( 66.20000000000000284, 71.98667160128370313, 3.500000001229034208 ) ) ;
#12250=CARTESIAN_POINT ( 'NONE',  ( 66.20000000000000284, 71.98667160128370313, 3.837500000000000799 ) ) ;
#12251=ORIENTED_EDGE ( 'NONE', *, *, #5108, .T. ) ;
#12254=CARTESIAN_POINT ( 'NONE',  ( 3.800000000000015365, 90.00000000000000000, 3.650000000000000355 ) ) ;
#12258=CARTESIAN_POINT ( 'NONE',  ( 60.63303222545420823, 111.5086687406912347, 2.829484441871016109 ) ) ;
#12260=CARTESIAN_POINT ( 'NONE',  ( 66.44356964375000985, 71.84604660189820891, 3.696875000614517237 ) ) ;
#12262=EDGE_CURVE ( 'NONE', #193, #5275, #6340, .T. ) ;
#12266=DIRECTION ( 'NONE',  ( -0.000000000000000000, -0.000000000000000000, -1.000000000000000000 ) ) ;
#12268=DIRECTION ( 'NONE',  ( -0.000000000000000000, -1.000000000000000000, -0.000000000000000000 ) ) ;
#12275=EDGE_CURVE ( 'NONE', #2032, #10118, #2978, .T. ) ;
#12280=DIRECTION ( 'NONE',  ( 1.000000000000000000, 0.000000000000000000, 0.000000000000000000 ) ) ;
#12283=DIRECTION ( 'NONE',  ( -0.000000000000000000, -0.000000000000000000, -1.000000000000000000 ) ) ;
#12284=ORIENTED_EDGE ( 'NONE', *, *, #11517, .T. ) ;
#12286=DIRECTION ( 'NONE',  ( -1.445602896647339656E-17, 0.000000000000000000, -1.000000000000000000 ) ) ;
#12302=EDGE_CURVE ( 'NONE', #5275, #5282, #3266, .T. ) ;
#12308=EDGE_CURVE ( 'NONE', #8376, #2989, #9440, .T. ) ;
#12312=CARTESIAN_POINT ( 'NONE',  ( 50.72178482187499071, 117.2309300971526937, 4.259375000614517681 ) ) ;
#12316=CARTESIAN_POINT ( 'NONE',  ( 50.60000000000001563, 62.98000740192552627, 3.800000000000000266 ) ) ;
#12317=PRODUCT_DEFINITION_SHAPE ( 'NONE', 'NONE',  #10165 ) ;
#12323=CARTESIAN_POINT ( 'NONE',  ( 64.54728993811707483, 100.7543353701752125, 2.858851390224067313 ) ) ;
#12326=CARTESIAN_POINT ( 'NONE',  ( 40.00000000000000000, 0.000000000000000000, -10.00000000000000000 ) ) ;
#12327=VECTOR ( 'NONE', #6578, 1000.000000000000000 ) ;
#12328=FACE_BOUND ( 'NONE', #5635, .T. ) ;
#12329=FACE_OUTER_BOUND ( 'NONE', #6074, .T. ) ;
#12330=LINE ( 'NONE', #9051, #1130 ) ;
#12342=CARTESIAN_POINT ( 'NONE',  ( 0.000000000000000000, 0.000000000000000000, -10.00000000000000000 ) ) ;
#12367=EDGE_LOOP ( 'NONE', ( #5160, #2944, #12739, #1420 ) ) ;
#12374=FACE_OUTER_BOUND ( 'NONE', #8024, .T. ) ;
#12376=CARTESIAN_POINT ( 'NONE',  ( 50.00000000000000000, 121.2009999999999934, 1.500000000000001332 ) ) ;
#12382=CARTESIAN_POINT ( 'NONE',  ( 50.72178482187501203, 62.76906990284730625, 4.559375000614517504 ) ) ;
#12392=CARTESIAN_POINT ( 'NONE',  ( 19.40000000000000924, 117.0199925980744666, 4.924999999999999822 ) ) ;
#12400=AXIS2_PLACEMENT_3D ( 'NONE', #12148, #10112, #12280 ) ;
#12415=EDGE_LOOP ( 'NONE', ( #11109, #2084 ) ) ;
#12432=ORIENTED_EDGE ( 'NONE', *, *, #12433, .T. ) ;
#12433=EDGE_CURVE ( 'NONE', #10547, #3551, #7783, .T. ) ;
#12436=ORIENTED_EDGE ( 'NONE', *, *, #5039, .F. ) ;
#12438=CARTESIAN_POINT ( 'NONE',  ( 50.59999999999999432, 117.0199925980744666, 3.162500001229034741 ) ) ;
#12441=ORIENTED_EDGE ( 'NONE', *, *, #11078, .F. ) ;
#12442=CARTESIAN_POINT ( 'NONE',  ( 19.40000000000002700, 62.98000740192551206, 4.287500001229034297 ) ) ;
#12452=CARTESIAN_POINT ( 'NONE',  ( 35.00000000000000000, 126.3079067962036106, 3.396875000614517415 ) ) ;
#12466=EDGE_CURVE ( 'NONE', #1104, #6338, #10913, .T. ) ;
#12468=CARTESIAN_POINT ( 'NONE',  ( 65.19999999999998863, 90.00000000000000000, -5.000000000000000000 ) ) ;
#12472=DIRECTION ( 'NONE',  ( 0.000000000000000000, -0.000000000000000000, 1.000000000000000000 ) ) ;
#12474=DIRECTION ( 'NONE',  ( -0.000000000000000000, -1.000000000000000000, -0.000000000000000000 ) ) ;
#12475=EDGE_CURVE ( 'NONE', #7686, #108, #12620, .T. ) ;
#12481=DIRECTION ( 'NONE',  ( -0.000000000000000000, -0.000000000000000000, 1.000000000000000000 ) ) ;
#12487=CARTESIAN_POINT ( 'NONE',  ( 25.00000000000000355, 0.000000000000000000, 5.750000000000000000 ) ) ;
#12492=DIRECTION ( 'NONE',  ( -0.000000000000000000, -0.000000000000000000, -1.000000000000000000 ) ) ;
#12494=ORIENTED_EDGE ( 'NONE', *, *, #12262, .T. ) ;
#12501=ORIENTED_EDGE ( 'NONE', *, *, #5678, .T. ) ;
#12510=CARTESIAN_POINT ( 'NONE',  ( 19.40000000000002700, 62.98000740192551206, 2.937500001229034208 ) ) ;
#12526=DIRECTION ( 'NONE',  ( -0.000000000000000000, -0.000000000000000000, -1.000000000000000000 ) ) ;
#12533=VERTEX_POINT ( 'NONE', #897 ) ;
#12545=CARTESIAN_POINT ( 'NONE',  ( 30.00000000000000711, 2.000000000000000000, 10.00000000000000000 ) ) ;
#12547=ORIENTED_EDGE ( 'NONE', *, *, #9870, .F. ) ;
#12549=EDGE_CURVE ( 'NONE', #10547, #11451, #11899, .T. ) ;
#12565=EDGE_LOOP ( 'NONE', ( #5786, #11134, #9789, #11991 ) ) ;
#12570=ORIENTED_EDGE ( 'NONE', *, *, #2926, .F. ) ;
#12577=CARTESIAN_POINT ( 'NONE',  ( 19.27821517812500574, 117.2309300971526937, 2.984375000614517326 ) ) ;
#12582=ORIENTED_EDGE ( 'NONE', *, *, #1437, .F. ) ;
#12606=PLANE ( 'NONE',  #91 ) ;
#12607=CARTESIAN_POINT ( 'NONE',  ( 66.44356964375000985, 71.84604660189820891, 3.190625000614517592 ) ) ;
#12617=DIRECTION ( 'NONE',  ( 0.000000000000000000, 0.000000000000000000, 1.000000000000000000 ) ) ;
#12620=( BOUNDED_CURVE ( )  B_SPLINE_CURVE ( 2, ( #5693, #514, #5562, #12028, #6003, #9868, #4054 ),
 .UNSPECIFIED., .F., .F. ) 
 B_SPLINE_CURVE_WITH_KNOTS ( ( 3, 2, 2, 3 ),
 ( 0.3000000000000002109, 0.3333333333333334259, 0.3666666666666666963, 0.3999999999999999667 ),
 .UNSPECIFIED. ) 
 CURVE ( )  GEOMETRIC_REPRESENTATION_ITEM ( )  RATIONAL_B_SPLINE_CURVE ( ( 0.9999999999999991118, 0.8660254037844395958, 1.000000000000000000, 0.8660254037844387076, 1.000000000000000000, 0.8660254037844389297, 0.9999999999999997780 ) ) 
 REPRESENTATION_ITEM ( '' )  );
#12624=VERTEX_POINT ( 'NONE', #1421 ) ;
#12640=CARTESIAN_POINT ( 'NONE',  ( 66.19999999999998863, 90.00000000000000000, 4.774999999999999467 ) ) ;
#12642=EDGE_CURVE ( 'NONE', #4450, #11781, #10777, .T. ) ;
#12647=ORIENTED_EDGE ( 'NONE', *, *, #9434, .T. ) ;
#12648=VECTOR ( 'NONE', #920, 1000.000000000000000 ) ;
#12649=CARTESIAN_POINT ( 'NONE',  ( 50.59999999999999432, 117.0199925980744666, 3.950000000000000178 ) ) ;
#12652=CARTESIAN_POINT ( 'NONE',  ( 66.44356964374998142, 108.1539533981018053, 3.265625000614516882 ) ) ;
#12654=DIRECTION ( 'NONE',  ( -1.000000000000000000, 0.000000000000000000, 0.000000000000000000 ) ) ;
#12660=DIRECTION ( 'NONE',  ( 0.8660254037844400399, 0.000000000000000000, -0.4999999999999975575 ) ) ;
#12661=CIRCLE ( 'NONE', #8690, 1.599999999999990319 ) ;
#12662=CARTESIAN_POINT ( 'NONE',  ( 3.556430356250028790, 71.84604660189818048, 3.996875000614517059 ) ) ;
#12665=AXIS2_PLACEMENT_3D ( 'NONE', #704, #11703, #2751 ) ;
#12667=EDGE_LOOP ( 'NONE', ( #5672, #2566, #3071, #4955, #7924, #7729, #844, #10119 ) ) ;
#12670=VECTOR ( 'NONE', #3862, 1000.000000000000000 ) ;
#12672=CARTESIAN_POINT ( 'NONE',  ( 17.66025403784438197, 77.14656965084323303, -1.000000000000000000 ) ) ;
#12682=DIRECTION ( 'NONE',  ( -1.000000000000000000, 0.000000000000000000, 0.000000000000000000 ) ) ;
#12686=ORIENTED_EDGE ( 'NONE', *, *, #5837, .F. ) ;
#12687=LINE ( 'NONE', #11637, #8045 ) ;
#12698=DIRECTION ( 'NONE',  ( -0.000000000000000000, -0.000000000000000000, -1.000000000000000000 ) ) ;
#12711=CARTESIAN_POINT ( 'NONE',  ( 66.44356964374999563, 90.00000000000000000, 3.678125000614516971 ) ) ;
#12712=EDGE_CURVE ( 'NONE', #7376, #10818, #61, .T. ) ;
#12722=CARTESIAN_POINT ( 'NONE',  ( 45.00000000000000000, 2.000000000000000000, 7.349999999999994316 ) ) ;
#12723=CARTESIAN_POINT ( 'NONE',  ( 19.27821517812500574, 117.2309300971526937, 2.984375000614517326 ) ) ;
#12725=VECTOR ( 'NONE', #8401, 1000.000000000000000 ) ;
#12733=FACE_OUTER_BOUND ( 'NONE', #9081, .T. ) ;
#12735=DIRECTION ( 'NONE',  ( -0.000000000000000000, -0.000000000000000000, -1.000000000000000000 ) ) ;
#12736=CARTESIAN_POINT ( 'NONE',  ( 3.556430356250028790, 71.84604660189818048, 4.390625000614517326 ) ) ;
#12739=ORIENTED_EDGE ( 'NONE', *, *, #7265, .F. ) ;
#12750=EDGE_LOOP ( 'NONE', ( #7960, #11457, #5899, #26 ) ) ;
#12752=PLANE ( 'NONE',  #12952 ) ;
#12762=EDGE_CURVE ( 'NONE', #9386, #9145, #7156, .T. ) ;
#12766=FACE_BOUND ( 'NONE', #11902, .T. ) ;
#12770=ORIENTED_EDGE ( 'NONE', *, *, #9603, .F. ) ;
#12774=CARTESIAN_POINT ( 'NONE',  ( 50.72178482187501203, 62.76906990284730625, 3.603125000614517681 ) ) ;
#12776=CIRCLE ( 'NONE', #3381, 1.599999999999986766 ) ;
#12785=CARTESIAN_POINT ( 'NONE',  ( 3.556430356250028790, 71.84604660189818048, 4.446875000614517681 ) ) ;
#12786=EDGE_LOOP ( 'NONE', ( #8650, #2144, #2009, #2345 ) ) ;
#12788=CARTESIAN_POINT ( 'NONE',  ( 35.00000000000000000, 126.0266567974326222, 3.650000001229033675 ) ) ;
#12795=CARTESIAN_POINT ( 'NONE',  ( 66.44356964375000985, 71.84604660189820891, 3.640625000614517326 ) ) ;
#12803=CARTESIAN_POINT ( 'NONE',  ( 25.00000000000000355, 0.000000000000000000, 5.750000000000000000 ) ) ;
#12810=ORIENTED_EDGE ( 'NONE', *, *, #3712, .T. ) ;
#12811=VECTOR ( 'NONE', #4828, 1000.000000000000000 ) ;
#12815=VERTEX_POINT ( 'NONE', #4571 ) ;
#12831=AXIS2_PLACEMENT_3D ( 'NONE', #2980, #6964, #10949 ) ;
#12836=CARTESIAN_POINT ( 'NONE',  ( 50.72178482187501203, 62.76906990284730625, 3.153125000614517504 ) ) ;
#12839=VERTEX_POINT ( 'NONE', #5673 ) ;
#12845=( BOUNDED_CURVE ( )  B_SPLINE_CURVE ( 2, ( #5193, #206, #8660, #2714, #5448, #7677, #11665 ),
 .UNSPECIFIED., .F., .F. ) 
 B_SPLINE_CURVE_WITH_KNOTS ( ( 3, 2, 2, 3 ),
 ( 0.3000000000000002109, 0.3333333333333334259, 0.3666666666666666963, 0.3999999999999999667 ),
 .UNSPECIFIED. ) 
 CURVE ( )  GEOMETRIC_REPRESENTATION_ITEM ( )  RATIONAL_B_SPLINE_CURVE ( ( 0.9999999999999991118, 0.8660254037844395958, 1.000000000000000000, 0.8660254037844387076, 1.000000000000000000, 0.8660254037844389297, 0.9999999999999997780 ) ) 
 REPRESENTATION_ITEM ( '' )  );
#12850=CARTESIAN_POINT ( 'NONE',  ( 66.44356964374999563, 90.00000000000000000, 3.734375000614516882 ) ) ;
#12860=CARTESIAN_POINT ( 'NONE',  ( 64.39470308771993246, 100.6987976320522336, 2.952601389814389687 ) ) ;
#12867=ORIENTED_EDGE ( 'NONE', *, *, #8400, .F. ) ;
#12873=CARTESIAN_POINT ( 'NONE',  ( 19.40000000000000924, 117.0199925980744666, 3.575000000000000178 ) ) ;
#12885=VECTOR ( 'NONE', #2864, 1000.000000000000000 ) ;
#12886=DIRECTION ( 'NONE',  ( 1.000000000000000000, 0.000000000000000000, -1.445602896647339656E-17 ) ) ;
#12897=ORIENTED_EDGE ( 'NONE', *, *, #5464, .T. ) ;
#12902=CARTESIAN_POINT ( 'NONE',  ( 64.54728994471078352, 100.7543353520590870, 2.802601390178781404 ) ) ;
#12910=VERTEX_POINT ( 'NONE', #11022 ) ;
#12914=CARTESIAN_POINT ( 'NONE',  ( 66.44356964374999563, 90.00000000000000000, 4.184375000614516615 ) ) ;
#12925=AXIS2_PLACEMENT_3D ( 'NONE', #4540, #11465, #2452 ) ;
#12933=CIRCLE ( 'NONE', #9376, 30.19999999999999218 ) ;
#12935=CARTESIAN_POINT ( 'NONE',  ( 64.31840955652153013, 100.6710290542226431, 2.929163888449521025 ) ) ;
#12939=LINE ( 'NONE', #2082, #9717 ) ;
#12942=CIRCLE ( 'NONE', #5000, 31.19999999999999218 ) ;
#12947=EDGE_CURVE ( 'NONE', #1634, #10264, #2931, .T. ) ;
#12950=FACE_OUTER_BOUND ( 'NONE', #8638, .T. ) ;
#12951=ORIENTED_EDGE ( 'NONE', *, *, #2336, .F. ) ;
#12952=AXIS2_PLACEMENT_3D ( 'NONE', #8697, #958, #2939 ) ;
#13010=COLOUR_RGB('Off White',0.89,0.88,0.83);
#13011=FILL_AREA_STYLE_COLOUR('',#13010);
#13012=FILL_AREA_STYLE('',(#13011));
#13013=SURFACE_STYLE_FILL_AREA(#13012);
#13014=SURFACE_SIDE_STYLE('',(#13013));
#13015=SURFACE_STYLE_USAGE(.BOTH.,#13014);
#13016=PRESENTATION_STYLE_ASSIGNMENT((#13015));
ENDSEC;
END-ISO-10303-21;
